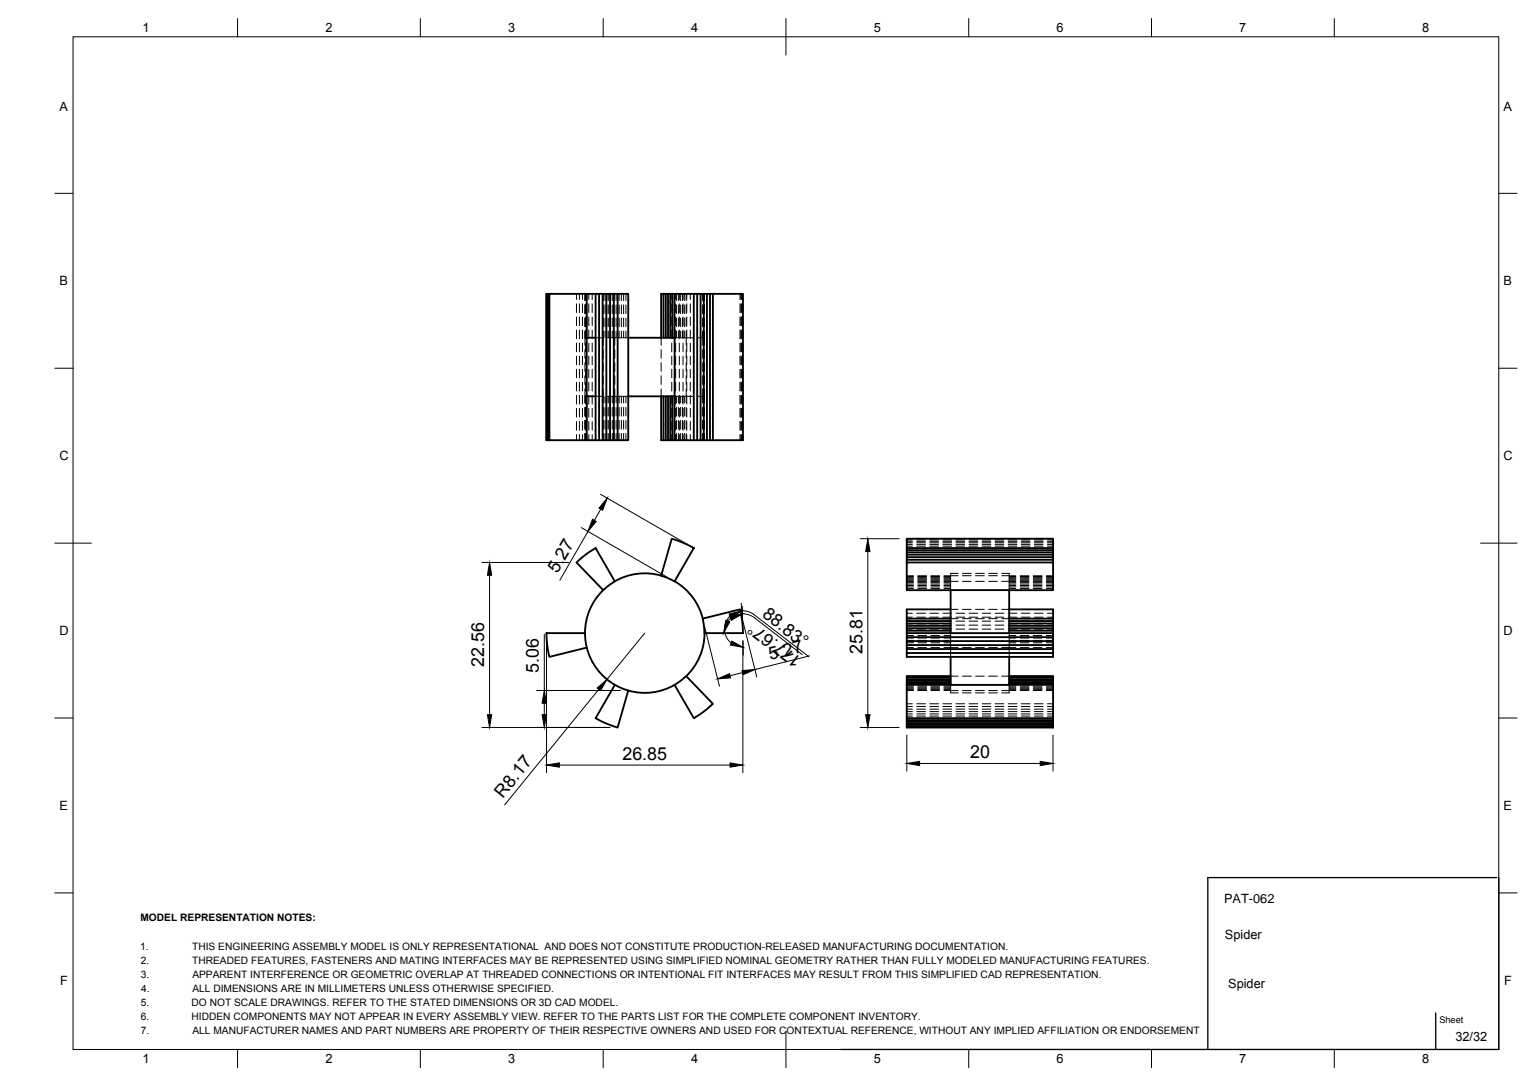
ISO-10303-21;
HEADER;
/* Generated by software containing ST-Developer
 * from STEP Tools, Inc. (www.steptools.com) 
 */

FILE_DESCRIPTION(
/* description */ ('Jaw-coupled motor to shaft test stand'),
/* implementation_level */ '2;1');

FILE_NAME(
/* name */ 'Spider.step',
/* time_stamp */ '2026-10-27T10:46:06-07:00',
/* author */ (''),
/* organization */ (''),
/* preprocessor_version */ 'ST-DEVELOPER v20.2',
/* originating_system */ 'Autodesk Translation Framework v15.17.0.0',
/* authorisation */ '');

FILE_SCHEMA (('AUTOMOTIVE_DESIGN { 1 0 10303 214 3 1 1 }'));
ENDSEC;

DATA;
#10=MECHANICAL_DESIGN_GEOMETRIC_PRESENTATION_REPRESENTATION('',(#369),#19361);
#304=SHAPE_REPRESENTATION_RELATIONSHIP('SRR','None',#19521,#336);
#336=ADVANCED_BREP_SHAPE_REPRESENTATION('',(#400),#19357);
#369=STYLED_ITEM('',(#19739),#400);
#400=MANIFOLD_SOLID_BREP('Body1',#11015);
#860=PLANE('',#12101);
#861=PLANE('',#12120);
#862=PLANE('',#12121);
#863=PLANE('',#12122);
#864=PLANE('',#12123);
#865=PLANE('',#12124);
#866=PLANE('',#12125);
#867=PLANE('',#12126);
#868=PLANE('',#12127);
#869=PLANE('',#12128);
#870=PLANE('',#12129);
#871=PLANE('',#12130);
#872=PLANE('',#12131);
#873=PLANE('',#12132);
#874=PLANE('',#12133);
#875=PLANE('',#12134);
#876=PLANE('',#12135);
#877=PLANE('',#12136);
#878=PLANE('',#12137);
#879=PLANE('',#12138);
#880=PLANE('',#12139);
#881=PLANE('',#12140);
#882=PLANE('',#12141);
#883=PLANE('',#12142);
#884=PLANE('',#12143);
#885=PLANE('',#12144);
#886=PLANE('',#12145);
#887=PLANE('',#12146);
#888=PLANE('',#12147);
#889=PLANE('',#12148);
#890=PLANE('',#12149);
#891=PLANE('',#12150);
#892=PLANE('',#12151);
#893=PLANE('',#12152);
#894=PLANE('',#12153);
#895=PLANE('',#12154);
#896=PLANE('',#12155);
#897=PLANE('',#12156);
#898=PLANE('',#12157);
#899=PLANE('',#12158);
#900=PLANE('',#12159);
#901=PLANE('',#12160);
#902=PLANE('',#12161);
#903=PLANE('',#12162);
#904=PLANE('',#12163);
#905=PLANE('',#12164);
#906=PLANE('',#12165);
#907=PLANE('',#12166);
#908=PLANE('',#12167);
#909=PLANE('',#12168);
#910=PLANE('',#12169);
#911=PLANE('',#12170);
#912=PLANE('',#12171);
#913=PLANE('',#12172);
#914=PLANE('',#12173);
#915=PLANE('',#12174);
#916=PLANE('',#12175);
#917=PLANE('',#12176);
#918=PLANE('',#12177);
#919=PLANE('',#12178);
#920=PLANE('',#12179);
#921=PLANE('',#12180);
#922=PLANE('',#12181);
#923=PLANE('',#12182);
#924=PLANE('',#12183);
#925=PLANE('',#12184);
#926=PLANE('',#12185);
#927=PLANE('',#12186);
#928=PLANE('',#12187);
#929=PLANE('',#12188);
#930=PLANE('',#12189);
#931=PLANE('',#12190);
#932=PLANE('',#12191);
#933=PLANE('',#12192);
#934=PLANE('',#12193);
#935=PLANE('',#12194);
#936=PLANE('',#12195);
#937=PLANE('',#12196);
#938=PLANE('',#12197);
#939=PLANE('',#12198);
#940=PLANE('',#12199);
#941=PLANE('',#12200);
#942=PLANE('',#12201);
#943=PLANE('',#12202);
#944=PLANE('',#12203);
#945=PLANE('',#12204);
#946=PLANE('',#12205);
#947=PLANE('',#12206);
#948=PLANE('',#12207);
#949=PLANE('',#12208);
#950=PLANE('',#12209);
#951=PLANE('',#12210);
#952=PLANE('',#12211);
#953=PLANE('',#12212);
#954=PLANE('',#12213);
#955=PLANE('',#12214);
#956=PLANE('',#12215);
#957=PLANE('',#12216);
#958=PLANE('',#12217);
#959=PLANE('',#12218);
#960=PLANE('',#12219);
#961=PLANE('',#12220);
#962=PLANE('',#12221);
#963=PLANE('',#12222);
#964=PLANE('',#12223);
#965=PLANE('',#12224);
#966=PLANE('',#12225);
#967=PLANE('',#12226);
#968=PLANE('',#12227);
#969=PLANE('',#12228);
#970=PLANE('',#12229);
#971=PLANE('',#12230);
#972=PLANE('',#12231);
#973=PLANE('',#12232);
#974=PLANE('',#12233);
#975=PLANE('',#12234);
#976=PLANE('',#12235);
#977=PLANE('',#12236);
#978=PLANE('',#12237);
#979=PLANE('',#12238);
#980=PLANE('',#12239);
#981=PLANE('',#12240);
#982=PLANE('',#12241);
#983=PLANE('',#12242);
#984=PLANE('',#12243);
#985=PLANE('',#12244);
#986=PLANE('',#12245);
#987=PLANE('',#12246);
#988=PLANE('',#12247);
#989=PLANE('',#12248);
#990=PLANE('',#12249);
#991=PLANE('',#12250);
#992=PLANE('',#12251);
#993=PLANE('',#12252);
#1459=FACE_OUTER_BOUND('',#2190,.T.);
#1460=FACE_OUTER_BOUND('',#2191,.T.);
#1461=FACE_OUTER_BOUND('',#2192,.T.);
#1462=FACE_OUTER_BOUND('',#2193,.T.);
#1463=FACE_OUTER_BOUND('',#2194,.T.);
#1464=FACE_OUTER_BOUND('',#2195,.T.);
#1465=FACE_OUTER_BOUND('',#2196,.T.);
#1466=FACE_OUTER_BOUND('',#2197,.T.);
#1467=FACE_OUTER_BOUND('',#2198,.T.);
#1468=FACE_OUTER_BOUND('',#2199,.T.);
#1469=FACE_OUTER_BOUND('',#2200,.T.);
#1470=FACE_OUTER_BOUND('',#2201,.T.);
#1471=FACE_OUTER_BOUND('',#2202,.T.);
#1472=FACE_OUTER_BOUND('',#2203,.T.);
#1473=FACE_OUTER_BOUND('',#2204,.T.);
#1474=FACE_OUTER_BOUND('',#2205,.T.);
#1475=FACE_OUTER_BOUND('',#2206,.T.);
#1476=FACE_OUTER_BOUND('',#2207,.T.);
#1477=FACE_OUTER_BOUND('',#2208,.T.);
#1478=FACE_OUTER_BOUND('',#2209,.T.);
#1479=FACE_OUTER_BOUND('',#2210,.T.);
#1480=FACE_OUTER_BOUND('',#2211,.T.);
#1481=FACE_OUTER_BOUND('',#2212,.T.);
#1482=FACE_OUTER_BOUND('',#2213,.T.);
#1483=FACE_OUTER_BOUND('',#2214,.T.);
#1484=FACE_OUTER_BOUND('',#2215,.T.);
#1485=FACE_OUTER_BOUND('',#2216,.T.);
#1486=FACE_OUTER_BOUND('',#2217,.T.);
#1487=FACE_OUTER_BOUND('',#2218,.T.);
#1488=FACE_OUTER_BOUND('',#2219,.T.);
#1489=FACE_OUTER_BOUND('',#2220,.T.);
#1490=FACE_OUTER_BOUND('',#2221,.T.);
#1491=FACE_OUTER_BOUND('',#2222,.T.);
#1492=FACE_OUTER_BOUND('',#2223,.T.);
#1493=FACE_OUTER_BOUND('',#2224,.T.);
#1494=FACE_OUTER_BOUND('',#2225,.T.);
#1495=FACE_OUTER_BOUND('',#2226,.T.);
#1496=FACE_OUTER_BOUND('',#2227,.T.);
#1497=FACE_OUTER_BOUND('',#2228,.T.);
#1498=FACE_OUTER_BOUND('',#2229,.T.);
#1499=FACE_OUTER_BOUND('',#2230,.T.);
#1500=FACE_OUTER_BOUND('',#2231,.T.);
#1501=FACE_OUTER_BOUND('',#2232,.T.);
#1502=FACE_OUTER_BOUND('',#2233,.T.);
#1503=FACE_OUTER_BOUND('',#2234,.T.);
#1504=FACE_OUTER_BOUND('',#2235,.T.);
#1505=FACE_OUTER_BOUND('',#2236,.T.);
#1506=FACE_OUTER_BOUND('',#2237,.T.);
#1507=FACE_OUTER_BOUND('',#2238,.T.);
#1508=FACE_OUTER_BOUND('',#2239,.T.);
#1509=FACE_OUTER_BOUND('',#2240,.T.);
#1510=FACE_OUTER_BOUND('',#2241,.T.);
#1511=FACE_OUTER_BOUND('',#2242,.T.);
#1512=FACE_OUTER_BOUND('',#2243,.T.);
#1513=FACE_OUTER_BOUND('',#2244,.T.);
#1514=FACE_OUTER_BOUND('',#2245,.T.);
#1515=FACE_OUTER_BOUND('',#2246,.T.);
#1516=FACE_OUTER_BOUND('',#2247,.T.);
#1517=FACE_OUTER_BOUND('',#2248,.T.);
#1518=FACE_OUTER_BOUND('',#2249,.T.);
#1519=FACE_OUTER_BOUND('',#2250,.T.);
#1520=FACE_OUTER_BOUND('',#2251,.T.);
#1521=FACE_OUTER_BOUND('',#2252,.T.);
#1522=FACE_OUTER_BOUND('',#2253,.T.);
#1523=FACE_OUTER_BOUND('',#2254,.T.);
#1524=FACE_OUTER_BOUND('',#2255,.T.);
#1525=FACE_OUTER_BOUND('',#2256,.T.);
#1526=FACE_OUTER_BOUND('',#2257,.T.);
#1527=FACE_OUTER_BOUND('',#2258,.T.);
#1528=FACE_OUTER_BOUND('',#2259,.T.);
#1529=FACE_OUTER_BOUND('',#2260,.T.);
#1530=FACE_OUTER_BOUND('',#2261,.T.);
#1531=FACE_OUTER_BOUND('',#2262,.T.);
#1532=FACE_OUTER_BOUND('',#2263,.T.);
#1533=FACE_OUTER_BOUND('',#2264,.T.);
#1534=FACE_OUTER_BOUND('',#2265,.T.);
#1535=FACE_OUTER_BOUND('',#2266,.T.);
#1536=FACE_OUTER_BOUND('',#2267,.T.);
#1537=FACE_OUTER_BOUND('',#2268,.T.);
#1538=FACE_OUTER_BOUND('',#2269,.T.);
#1539=FACE_OUTER_BOUND('',#2270,.T.);
#1540=FACE_OUTER_BOUND('',#2271,.T.);
#1541=FACE_OUTER_BOUND('',#2272,.T.);
#1542=FACE_OUTER_BOUND('',#2273,.T.);
#1543=FACE_OUTER_BOUND('',#2274,.T.);
#1544=FACE_OUTER_BOUND('',#2275,.T.);
#1545=FACE_OUTER_BOUND('',#2276,.T.);
#1546=FACE_OUTER_BOUND('',#2277,.T.);
#1547=FACE_OUTER_BOUND('',#2278,.T.);
#1548=FACE_OUTER_BOUND('',#2279,.T.);
#1549=FACE_OUTER_BOUND('',#2280,.T.);
#1550=FACE_OUTER_BOUND('',#2281,.T.);
#1551=FACE_OUTER_BOUND('',#2282,.T.);
#1552=FACE_OUTER_BOUND('',#2283,.T.);
#1553=FACE_OUTER_BOUND('',#2284,.T.);
#1554=FACE_OUTER_BOUND('',#2285,.T.);
#1555=FACE_OUTER_BOUND('',#2286,.T.);
#1556=FACE_OUTER_BOUND('',#2287,.T.);
#1557=FACE_OUTER_BOUND('',#2288,.T.);
#1558=FACE_OUTER_BOUND('',#2289,.T.);
#1559=FACE_OUTER_BOUND('',#2290,.T.);
#1560=FACE_OUTER_BOUND('',#2291,.T.);
#1561=FACE_OUTER_BOUND('',#2292,.T.);
#1562=FACE_OUTER_BOUND('',#2293,.T.);
#1563=FACE_OUTER_BOUND('',#2294,.T.);
#1564=FACE_OUTER_BOUND('',#2295,.T.);
#1565=FACE_OUTER_BOUND('',#2296,.T.);
#1566=FACE_OUTER_BOUND('',#2297,.T.);
#1567=FACE_OUTER_BOUND('',#2298,.T.);
#1568=FACE_OUTER_BOUND('',#2299,.T.);
#1569=FACE_OUTER_BOUND('',#2300,.T.);
#1570=FACE_OUTER_BOUND('',#2301,.T.);
#1571=FACE_OUTER_BOUND('',#2302,.T.);
#1572=FACE_OUTER_BOUND('',#2303,.T.);
#1573=FACE_OUTER_BOUND('',#2304,.T.);
#1574=FACE_OUTER_BOUND('',#2305,.T.);
#1575=FACE_OUTER_BOUND('',#2306,.T.);
#1576=FACE_OUTER_BOUND('',#2307,.T.);
#1577=FACE_OUTER_BOUND('',#2308,.T.);
#1578=FACE_OUTER_BOUND('',#2309,.T.);
#1579=FACE_OUTER_BOUND('',#2310,.T.);
#1580=FACE_OUTER_BOUND('',#2311,.T.);
#1581=FACE_OUTER_BOUND('',#2312,.T.);
#1582=FACE_OUTER_BOUND('',#2313,.T.);
#1583=FACE_OUTER_BOUND('',#2314,.T.);
#1584=FACE_OUTER_BOUND('',#2315,.T.);
#1585=FACE_OUTER_BOUND('',#2316,.T.);
#1586=FACE_OUTER_BOUND('',#2317,.T.);
#1587=FACE_OUTER_BOUND('',#2318,.T.);
#1588=FACE_OUTER_BOUND('',#2319,.T.);
#1589=FACE_OUTER_BOUND('',#2320,.T.);
#1590=FACE_OUTER_BOUND('',#2321,.T.);
#1591=FACE_OUTER_BOUND('',#2322,.T.);
#1592=FACE_OUTER_BOUND('',#2323,.T.);
#1593=FACE_OUTER_BOUND('',#2324,.T.);
#1594=FACE_OUTER_BOUND('',#2325,.T.);
#1595=FACE_OUTER_BOUND('',#2326,.T.);
#1596=FACE_OUTER_BOUND('',#2327,.T.);
#1597=FACE_OUTER_BOUND('',#2328,.T.);
#1598=FACE_OUTER_BOUND('',#2329,.T.);
#2190=EDGE_LOOP('',(#9272,#9273,#9274,#9275,#9276,#9277,#9278,#9279,#9280,
#9281,#9282,#9283,#9284,#9285,#9286,#9287,#9288,#9289,#9290,#9291,#9292,
#9293,#9294,#9295,#9296,#9297,#9298,#9299,#9300,#9301,#9302,#9303,#9304,
#9305,#9306,#9307,#9308,#9309,#9310,#9311,#9312,#9313,#9314,#9315,#9316,
#9317,#9318,#9319,#9320,#9321,#9322,#9323,#9324,#9325));
#2191=EDGE_LOOP('',(#9326,#9327,#9328,#9329));
#2192=EDGE_LOOP('',(#9330,#9331,#9332,#9333));
#2193=EDGE_LOOP('',(#9334,#9335,#9336,#9337));
#2194=EDGE_LOOP('',(#9338,#9339,#9340,#9341));
#2195=EDGE_LOOP('',(#9342,#9343,#9344,#9345));
#2196=EDGE_LOOP('',(#9346,#9347,#9348,#9349));
#2197=EDGE_LOOP('',(#9350,#9351,#9352,#9353,#9354,#9355,#9356,#9357,#9358,
#9359,#9360,#9361,#9362,#9363,#9364,#9365,#9366,#9367,#9368,#9369,#9370,
#9371,#9372,#9373,#9374,#9375,#9376,#9377,#9378,#9379,#9380,#9381,#9382,
#9383,#9384,#9385,#9386,#9387,#9388,#9389,#9390,#9391,#9392,#9393,#9394,
#9395,#9396,#9397,#9398,#9399,#9400,#9401,#9402,#9403));
#2198=EDGE_LOOP('',(#9404,#9405,#9406,#9407,#9408,#9409,#9410,#9411));
#2199=EDGE_LOOP('',(#9412,#9413,#9414,#9415));
#2200=EDGE_LOOP('',(#9416,#9417,#9418,#9419));
#2201=EDGE_LOOP('',(#9420,#9421,#9422,#9423));
#2202=EDGE_LOOP('',(#9424,#9425,#9426,#9427));
#2203=EDGE_LOOP('',(#9428,#9429,#9430,#9431));
#2204=EDGE_LOOP('',(#9432,#9433,#9434,#9435));
#2205=EDGE_LOOP('',(#9436,#9437,#9438,#9439));
#2206=EDGE_LOOP('',(#9440,#9441,#9442,#9443,#9444,#9445,#9446,#9447,#9448,
#9449,#9450,#9451,#9452,#9453));
#2207=EDGE_LOOP('',(#9454,#9455,#9456,#9457));
#2208=EDGE_LOOP('',(#9458,#9459,#9460,#9461));
#2209=EDGE_LOOP('',(#9462,#9463,#9464,#9465));
#2210=EDGE_LOOP('',(#9466,#9467,#9468,#9469));
#2211=EDGE_LOOP('',(#9470,#9471,#9472,#9473));
#2212=EDGE_LOOP('',(#9474,#9475,#9476,#9477));
#2213=EDGE_LOOP('',(#9478,#9479,#9480,#9481));
#2214=EDGE_LOOP('',(#9482,#9483,#9484,#9485));
#2215=EDGE_LOOP('',(#9486,#9487,#9488,#9489));
#2216=EDGE_LOOP('',(#9490,#9491,#9492,#9493));
#2217=EDGE_LOOP('',(#9494,#9495,#9496,#9497));
#2218=EDGE_LOOP('',(#9498,#9499,#9500,#9501,#9502,#9503,#9504,#9505));
#2219=EDGE_LOOP('',(#9506,#9507,#9508,#9509,#9510,#9511,#9512,#9513,#9514,
#9515,#9516,#9517,#9518,#9519));
#2220=EDGE_LOOP('',(#9520,#9521,#9522,#9523,#9524,#9525,#9526,#9527));
#2221=EDGE_LOOP('',(#9528,#9529,#9530,#9531));
#2222=EDGE_LOOP('',(#9532,#9533,#9534,#9535));
#2223=EDGE_LOOP('',(#9536,#9537,#9538,#9539));
#2224=EDGE_LOOP('',(#9540,#9541,#9542,#9543));
#2225=EDGE_LOOP('',(#9544,#9545,#9546,#9547));
#2226=EDGE_LOOP('',(#9548,#9549,#9550,#9551));
#2227=EDGE_LOOP('',(#9552,#9553,#9554,#9555));
#2228=EDGE_LOOP('',(#9556,#9557,#9558,#9559,#9560,#9561,#9562,#9563,#9564,
#9565,#9566,#9567,#9568,#9569));
#2229=EDGE_LOOP('',(#9570,#9571,#9572,#9573));
#2230=EDGE_LOOP('',(#9574,#9575,#9576,#9577));
#2231=EDGE_LOOP('',(#9578,#9579,#9580,#9581));
#2232=EDGE_LOOP('',(#9582,#9583,#9584,#9585));
#2233=EDGE_LOOP('',(#9586,#9587,#9588,#9589));
#2234=EDGE_LOOP('',(#9590,#9591,#9592,#9593));
#2235=EDGE_LOOP('',(#9594,#9595,#9596,#9597));
#2236=EDGE_LOOP('',(#9598,#9599,#9600,#9601));
#2237=EDGE_LOOP('',(#9602,#9603,#9604,#9605));
#2238=EDGE_LOOP('',(#9606,#9607,#9608,#9609));
#2239=EDGE_LOOP('',(#9610,#9611,#9612,#9613));
#2240=EDGE_LOOP('',(#9614,#9615,#9616,#9617,#9618,#9619,#9620,#9621));
#2241=EDGE_LOOP('',(#9622,#9623,#9624,#9625,#9626,#9627,#9628,#9629,#9630,
#9631,#9632,#9633,#9634,#9635));
#2242=EDGE_LOOP('',(#9636,#9637,#9638,#9639,#9640,#9641,#9642,#9643));
#2243=EDGE_LOOP('',(#9644,#9645,#9646,#9647));
#2244=EDGE_LOOP('',(#9648,#9649,#9650,#9651));
#2245=EDGE_LOOP('',(#9652,#9653,#9654,#9655));
#2246=EDGE_LOOP('',(#9656,#9657,#9658,#9659));
#2247=EDGE_LOOP('',(#9660,#9661,#9662,#9663));
#2248=EDGE_LOOP('',(#9664,#9665,#9666,#9667));
#2249=EDGE_LOOP('',(#9668,#9669,#9670,#9671));
#2250=EDGE_LOOP('',(#9672,#9673,#9674,#9675,#9676,#9677,#9678,#9679,#9680,
#9681,#9682,#9683,#9684,#9685));
#2251=EDGE_LOOP('',(#9686,#9687,#9688,#9689));
#2252=EDGE_LOOP('',(#9690,#9691,#9692,#9693));
#2253=EDGE_LOOP('',(#9694,#9695,#9696,#9697));
#2254=EDGE_LOOP('',(#9698,#9699,#9700,#9701));
#2255=EDGE_LOOP('',(#9702,#9703,#9704,#9705));
#2256=EDGE_LOOP('',(#9706,#9707,#9708,#9709));
#2257=EDGE_LOOP('',(#9710,#9711,#9712,#9713));
#2258=EDGE_LOOP('',(#9714,#9715,#9716,#9717));
#2259=EDGE_LOOP('',(#9718,#9719,#9720,#9721));
#2260=EDGE_LOOP('',(#9722,#9723,#9724,#9725));
#2261=EDGE_LOOP('',(#9726,#9727,#9728,#9729));
#2262=EDGE_LOOP('',(#9730,#9731,#9732,#9733,#9734,#9735,#9736,#9737));
#2263=EDGE_LOOP('',(#9738,#9739,#9740,#9741,#9742,#9743,#9744,#9745,#9746,
#9747,#9748,#9749,#9750,#9751));
#2264=EDGE_LOOP('',(#9752,#9753,#9754,#9755,#9756,#9757,#9758,#9759));
#2265=EDGE_LOOP('',(#9760,#9761,#9762,#9763));
#2266=EDGE_LOOP('',(#9764,#9765,#9766,#9767));
#2267=EDGE_LOOP('',(#9768,#9769,#9770,#9771));
#2268=EDGE_LOOP('',(#9772,#9773,#9774,#9775));
#2269=EDGE_LOOP('',(#9776,#9777,#9778,#9779));
#2270=EDGE_LOOP('',(#9780,#9781,#9782,#9783));
#2271=EDGE_LOOP('',(#9784,#9785,#9786,#9787));
#2272=EDGE_LOOP('',(#9788,#9789,#9790,#9791,#9792,#9793,#9794,#9795,#9796,
#9797,#9798,#9799,#9800,#9801));
#2273=EDGE_LOOP('',(#9802,#9803,#9804,#9805));
#2274=EDGE_LOOP('',(#9806,#9807,#9808,#9809));
#2275=EDGE_LOOP('',(#9810,#9811,#9812,#9813));
#2276=EDGE_LOOP('',(#9814,#9815,#9816,#9817));
#2277=EDGE_LOOP('',(#9818,#9819,#9820,#9821));
#2278=EDGE_LOOP('',(#9822,#9823,#9824,#9825));
#2279=EDGE_LOOP('',(#9826,#9827,#9828,#9829));
#2280=EDGE_LOOP('',(#9830,#9831,#9832,#9833));
#2281=EDGE_LOOP('',(#9834,#9835,#9836,#9837));
#2282=EDGE_LOOP('',(#9838,#9839,#9840,#9841));
#2283=EDGE_LOOP('',(#9842,#9843,#9844,#9845));
#2284=EDGE_LOOP('',(#9846,#9847,#9848,#9849,#9850,#9851,#9852,#9853));
#2285=EDGE_LOOP('',(#9854,#9855,#9856,#9857,#9858,#9859,#9860,#9861,#9862,
#9863,#9864,#9865,#9866,#9867));
#2286=EDGE_LOOP('',(#9868,#9869,#9870,#9871,#9872,#9873,#9874,#9875));
#2287=EDGE_LOOP('',(#9876,#9877,#9878,#9879));
#2288=EDGE_LOOP('',(#9880,#9881,#9882,#9883));
#2289=EDGE_LOOP('',(#9884,#9885,#9886,#9887));
#2290=EDGE_LOOP('',(#9888,#9889,#9890,#9891));
#2291=EDGE_LOOP('',(#9892,#9893,#9894,#9895));
#2292=EDGE_LOOP('',(#9896,#9897,#9898,#9899));
#2293=EDGE_LOOP('',(#9900,#9901,#9902,#9903));
#2294=EDGE_LOOP('',(#9904,#9905,#9906,#9907,#9908,#9909,#9910,#9911,#9912,
#9913,#9914,#9915,#9916,#9917));
#2295=EDGE_LOOP('',(#9918,#9919,#9920,#9921));
#2296=EDGE_LOOP('',(#9922,#9923,#9924,#9925));
#2297=EDGE_LOOP('',(#9926,#9927,#9928,#9929));
#2298=EDGE_LOOP('',(#9930,#9931,#9932,#9933));
#2299=EDGE_LOOP('',(#9934,#9935,#9936,#9937));
#2300=EDGE_LOOP('',(#9938,#9939,#9940,#9941));
#2301=EDGE_LOOP('',(#9942,#9943,#9944,#9945));
#2302=EDGE_LOOP('',(#9946,#9947,#9948,#9949));
#2303=EDGE_LOOP('',(#9950,#9951,#9952,#9953));
#2304=EDGE_LOOP('',(#9954,#9955,#9956,#9957));
#2305=EDGE_LOOP('',(#9958,#9959,#9960,#9961));
#2306=EDGE_LOOP('',(#9962,#9963,#9964,#9965,#9966,#9967,#9968,#9969));
#2307=EDGE_LOOP('',(#9970,#9971,#9972,#9973,#9974,#9975,#9976,#9977,#9978,
#9979,#9980,#9981,#9982,#9983));
#2308=EDGE_LOOP('',(#9984,#9985,#9986,#9987,#9988,#9989,#9990,#9991));
#2309=EDGE_LOOP('',(#9992,#9993,#9994,#9995));
#2310=EDGE_LOOP('',(#9996,#9997,#9998,#9999));
#2311=EDGE_LOOP('',(#10000,#10001,#10002,#10003));
#2312=EDGE_LOOP('',(#10004,#10005,#10006,#10007));
#2313=EDGE_LOOP('',(#10008,#10009,#10010,#10011));
#2314=EDGE_LOOP('',(#10012,#10013,#10014,#10015));
#2315=EDGE_LOOP('',(#10016,#10017,#10018,#10019));
#2316=EDGE_LOOP('',(#10020,#10021,#10022,#10023,#10024,#10025,#10026,#10027,
#10028,#10029,#10030,#10031,#10032,#10033));
#2317=EDGE_LOOP('',(#10034,#10035,#10036,#10037));
#2318=EDGE_LOOP('',(#10038,#10039,#10040,#10041));
#2319=EDGE_LOOP('',(#10042,#10043,#10044,#10045));
#2320=EDGE_LOOP('',(#10046,#10047,#10048,#10049));
#2321=EDGE_LOOP('',(#10050,#10051,#10052,#10053));
#2322=EDGE_LOOP('',(#10054,#10055,#10056,#10057));
#2323=EDGE_LOOP('',(#10058,#10059,#10060,#10061));
#2324=EDGE_LOOP('',(#10062,#10063,#10064,#10065));
#2325=EDGE_LOOP('',(#10066,#10067,#10068,#10069));
#2326=EDGE_LOOP('',(#10070,#10071,#10072,#10073));
#2327=EDGE_LOOP('',(#10074,#10075,#10076,#10077));
#2328=EDGE_LOOP('',(#10078,#10079,#10080,#10081,#10082,#10083,#10084,#10085));
#2329=EDGE_LOOP('',(#10086,#10087,#10088,#10089,#10090,#10091,#10092,#10093,
#10094,#10095,#10096,#10097,#10098,#10099));
#3061=LINE('',#18255,#4214);
#3062=LINE('',#18257,#4215);
#3063=LINE('',#18259,#4216);
#3064=LINE('',#18261,#4217);
#3065=LINE('',#18263,#4218);
#3066=LINE('',#18265,#4219);
#3067=LINE('',#18267,#4220);
#3068=LINE('',#18269,#4221);
#3069=LINE('',#18273,#4222);
#3070=LINE('',#18275,#4223);
#3071=LINE('',#18277,#4224);
#3072=LINE('',#18279,#4225);
#3073=LINE('',#18281,#4226);
#3074=LINE('',#18283,#4227);
#3075=LINE('',#18285,#4228);
#3076=LINE('',#18287,#4229);
#3077=LINE('',#18291,#4230);
#3078=LINE('',#18293,#4231);
#3079=LINE('',#18295,#4232);
#3080=LINE('',#18297,#4233);
#3081=LINE('',#18299,#4234);
#3082=LINE('',#18301,#4235);
#3083=LINE('',#18303,#4236);
#3084=LINE('',#18305,#4237);
#3085=LINE('',#18309,#4238);
#3086=LINE('',#18311,#4239);
#3087=LINE('',#18313,#4240);
#3088=LINE('',#18315,#4241);
#3089=LINE('',#18317,#4242);
#3090=LINE('',#18319,#4243);
#3091=LINE('',#18321,#4244);
#3092=LINE('',#18323,#4245);
#3093=LINE('',#18327,#4246);
#3094=LINE('',#18329,#4247);
#3095=LINE('',#18331,#4248);
#3096=LINE('',#18333,#4249);
#3097=LINE('',#18335,#4250);
#3098=LINE('',#18337,#4251);
#3099=LINE('',#18339,#4252);
#3100=LINE('',#18341,#4253);
#3101=LINE('',#18345,#4254);
#3102=LINE('',#18347,#4255);
#3103=LINE('',#18349,#4256);
#3104=LINE('',#18351,#4257);
#3105=LINE('',#18353,#4258);
#3106=LINE('',#18355,#4259);
#3107=LINE('',#18357,#4260);
#3108=LINE('',#18359,#4261);
#3109=LINE('',#18363,#4262);
#3110=LINE('',#18366,#4263);
#3111=LINE('',#18369,#4264);
#3112=LINE('',#18372,#4265);
#3113=LINE('',#18375,#4266);
#3114=LINE('',#18378,#4267);
#3115=LINE('',#18381,#4268);
#3116=LINE('',#18383,#4269);
#3117=LINE('',#18387,#4270);
#3118=LINE('',#18389,#4271);
#3119=LINE('',#18393,#4272);
#3120=LINE('',#18395,#4273);
#3121=LINE('',#18399,#4274);
#3122=LINE('',#18401,#4275);
#3123=LINE('',#18403,#4276);
#3124=LINE('',#18405,#4277);
#3125=LINE('',#18407,#4278);
#3126=LINE('',#18409,#4279);
#3127=LINE('',#18411,#4280);
#3128=LINE('',#18413,#4281);
#3129=LINE('',#18414,#4282);
#3130=LINE('',#18416,#4283);
#3131=LINE('',#18418,#4284);
#3132=LINE('',#18420,#4285);
#3133=LINE('',#18422,#4286);
#3134=LINE('',#18424,#4287);
#3135=LINE('',#18426,#4288);
#3136=LINE('',#18428,#4289);
#3137=LINE('',#18429,#4290);
#3138=LINE('',#18431,#4291);
#3139=LINE('',#18433,#4292);
#3140=LINE('',#18435,#4293);
#3141=LINE('',#18437,#4294);
#3142=LINE('',#18439,#4295);
#3143=LINE('',#18441,#4296);
#3144=LINE('',#18443,#4297);
#3145=LINE('',#18444,#4298);
#3146=LINE('',#18446,#4299);
#3147=LINE('',#18448,#4300);
#3148=LINE('',#18450,#4301);
#3149=LINE('',#18452,#4302);
#3150=LINE('',#18454,#4303);
#3151=LINE('',#18456,#4304);
#3152=LINE('',#18458,#4305);
#3153=LINE('',#18459,#4306);
#3154=LINE('',#18461,#4307);
#3155=LINE('',#18463,#4308);
#3156=LINE('',#18465,#4309);
#3157=LINE('',#18467,#4310);
#3158=LINE('',#18469,#4311);
#3159=LINE('',#18471,#4312);
#3160=LINE('',#18473,#4313);
#3161=LINE('',#18474,#4314);
#3162=LINE('',#18476,#4315);
#3163=LINE('',#18478,#4316);
#3164=LINE('',#18480,#4317);
#3165=LINE('',#18482,#4318);
#3166=LINE('',#18484,#4319);
#3167=LINE('',#18486,#4320);
#3168=LINE('',#18487,#4321);
#3169=LINE('',#18490,#4322);
#3170=LINE('',#18492,#4323);
#3171=LINE('',#18494,#4324);
#3172=LINE('',#18496,#4325);
#3173=LINE('',#18497,#4326);
#3174=LINE('',#18500,#4327);
#3175=LINE('',#18501,#4328);
#3176=LINE('',#18504,#4329);
#3177=LINE('',#18505,#4330);
#3178=LINE('',#18508,#4331);
#3179=LINE('',#18509,#4332);
#3180=LINE('',#18512,#4333);
#3181=LINE('',#18513,#4334);
#3182=LINE('',#18516,#4335);
#3183=LINE('',#18517,#4336);
#3184=LINE('',#18520,#4337);
#3185=LINE('',#18521,#4338);
#3186=LINE('',#18524,#4339);
#3187=LINE('',#18525,#4340);
#3188=LINE('',#18529,#4341);
#3189=LINE('',#18531,#4342);
#3190=LINE('',#18533,#4343);
#3191=LINE('',#18535,#4344);
#3192=LINE('',#18537,#4345);
#3193=LINE('',#18538,#4346);
#3194=LINE('',#18540,#4347);
#3195=LINE('',#18542,#4348);
#3196=LINE('',#18544,#4349);
#3197=LINE('',#18546,#4350);
#3198=LINE('',#18548,#4351);
#3199=LINE('',#18549,#4352);
#3200=LINE('',#18551,#4353);
#3201=LINE('',#18552,#4354);
#3202=LINE('',#18554,#4355);
#3203=LINE('',#18556,#4356);
#3204=LINE('',#18558,#4357);
#3205=LINE('',#18562,#4358);
#3206=LINE('',#18563,#4359);
#3207=LINE('',#18566,#4360);
#3208=LINE('',#18567,#4361);
#3209=LINE('',#18570,#4362);
#3210=LINE('',#18571,#4363);
#3211=LINE('',#18574,#4364);
#3212=LINE('',#18575,#4365);
#3213=LINE('',#18578,#4366);
#3214=LINE('',#18579,#4367);
#3215=LINE('',#18582,#4368);
#3216=LINE('',#18583,#4369);
#3217=LINE('',#18585,#4370);
#3218=LINE('',#18589,#4371);
#3219=LINE('',#18591,#4372);
#3220=LINE('',#18593,#4373);
#3221=LINE('',#18595,#4374);
#3222=LINE('',#18596,#4375);
#3223=LINE('',#18599,#4376);
#3224=LINE('',#18600,#4377);
#3225=LINE('',#18603,#4378);
#3226=LINE('',#18604,#4379);
#3227=LINE('',#18607,#4380);
#3228=LINE('',#18608,#4381);
#3229=LINE('',#18611,#4382);
#3230=LINE('',#18612,#4383);
#3231=LINE('',#18615,#4384);
#3232=LINE('',#18616,#4385);
#3233=LINE('',#18619,#4386);
#3234=LINE('',#18620,#4387);
#3235=LINE('',#18623,#4388);
#3236=LINE('',#18624,#4389);
#3237=LINE('',#18628,#4390);
#3238=LINE('',#18630,#4391);
#3239=LINE('',#18632,#4392);
#3240=LINE('',#18634,#4393);
#3241=LINE('',#18636,#4394);
#3242=LINE('',#18637,#4395);
#3243=LINE('',#18639,#4396);
#3244=LINE('',#18641,#4397);
#3245=LINE('',#18643,#4398);
#3246=LINE('',#18645,#4399);
#3247=LINE('',#18647,#4400);
#3248=LINE('',#18648,#4401);
#3249=LINE('',#18650,#4402);
#3250=LINE('',#18651,#4403);
#3251=LINE('',#18653,#4404);
#3252=LINE('',#18655,#4405);
#3253=LINE('',#18657,#4406);
#3254=LINE('',#18661,#4407);
#3255=LINE('',#18662,#4408);
#3256=LINE('',#18665,#4409);
#3257=LINE('',#18666,#4410);
#3258=LINE('',#18669,#4411);
#3259=LINE('',#18670,#4412);
#3260=LINE('',#18673,#4413);
#3261=LINE('',#18674,#4414);
#3262=LINE('',#18677,#4415);
#3263=LINE('',#18678,#4416);
#3264=LINE('',#18681,#4417);
#3265=LINE('',#18682,#4418);
#3266=LINE('',#18684,#4419);
#3267=LINE('',#18688,#4420);
#3268=LINE('',#18690,#4421);
#3269=LINE('',#18692,#4422);
#3270=LINE('',#18694,#4423);
#3271=LINE('',#18695,#4424);
#3272=LINE('',#18698,#4425);
#3273=LINE('',#18699,#4426);
#3274=LINE('',#18702,#4427);
#3275=LINE('',#18703,#4428);
#3276=LINE('',#18706,#4429);
#3277=LINE('',#18707,#4430);
#3278=LINE('',#18710,#4431);
#3279=LINE('',#18711,#4432);
#3280=LINE('',#18714,#4433);
#3281=LINE('',#18715,#4434);
#3282=LINE('',#18718,#4435);
#3283=LINE('',#18719,#4436);
#3284=LINE('',#18722,#4437);
#3285=LINE('',#18723,#4438);
#3286=LINE('',#18727,#4439);
#3287=LINE('',#18729,#4440);
#3288=LINE('',#18731,#4441);
#3289=LINE('',#18733,#4442);
#3290=LINE('',#18735,#4443);
#3291=LINE('',#18736,#4444);
#3292=LINE('',#18738,#4445);
#3293=LINE('',#18740,#4446);
#3294=LINE('',#18742,#4447);
#3295=LINE('',#18744,#4448);
#3296=LINE('',#18746,#4449);
#3297=LINE('',#18747,#4450);
#3298=LINE('',#18749,#4451);
#3299=LINE('',#18750,#4452);
#3300=LINE('',#18752,#4453);
#3301=LINE('',#18754,#4454);
#3302=LINE('',#18756,#4455);
#3303=LINE('',#18760,#4456);
#3304=LINE('',#18761,#4457);
#3305=LINE('',#18764,#4458);
#3306=LINE('',#18765,#4459);
#3307=LINE('',#18768,#4460);
#3308=LINE('',#18769,#4461);
#3309=LINE('',#18772,#4462);
#3310=LINE('',#18773,#4463);
#3311=LINE('',#18776,#4464);
#3312=LINE('',#18777,#4465);
#3313=LINE('',#18780,#4466);
#3314=LINE('',#18781,#4467);
#3315=LINE('',#18783,#4468);
#3316=LINE('',#18787,#4469);
#3317=LINE('',#18789,#4470);
#3318=LINE('',#18791,#4471);
#3319=LINE('',#18793,#4472);
#3320=LINE('',#18794,#4473);
#3321=LINE('',#18797,#4474);
#3322=LINE('',#18798,#4475);
#3323=LINE('',#18801,#4476);
#3324=LINE('',#18802,#4477);
#3325=LINE('',#18805,#4478);
#3326=LINE('',#18806,#4479);
#3327=LINE('',#18809,#4480);
#3328=LINE('',#18810,#4481);
#3329=LINE('',#18813,#4482);
#3330=LINE('',#18814,#4483);
#3331=LINE('',#18817,#4484);
#3332=LINE('',#18818,#4485);
#3333=LINE('',#18821,#4486);
#3334=LINE('',#18822,#4487);
#3335=LINE('',#18826,#4488);
#3336=LINE('',#18828,#4489);
#3337=LINE('',#18830,#4490);
#3338=LINE('',#18832,#4491);
#3339=LINE('',#18834,#4492);
#3340=LINE('',#18835,#4493);
#3341=LINE('',#18837,#4494);
#3342=LINE('',#18839,#4495);
#3343=LINE('',#18841,#4496);
#3344=LINE('',#18843,#4497);
#3345=LINE('',#18845,#4498);
#3346=LINE('',#18846,#4499);
#3347=LINE('',#18848,#4500);
#3348=LINE('',#18849,#4501);
#3349=LINE('',#18851,#4502);
#3350=LINE('',#18853,#4503);
#3351=LINE('',#18855,#4504);
#3352=LINE('',#18859,#4505);
#3353=LINE('',#18860,#4506);
#3354=LINE('',#18863,#4507);
#3355=LINE('',#18864,#4508);
#3356=LINE('',#18867,#4509);
#3357=LINE('',#18868,#4510);
#3358=LINE('',#18871,#4511);
#3359=LINE('',#18872,#4512);
#3360=LINE('',#18875,#4513);
#3361=LINE('',#18876,#4514);
#3362=LINE('',#18879,#4515);
#3363=LINE('',#18880,#4516);
#3364=LINE('',#18882,#4517);
#3365=LINE('',#18886,#4518);
#3366=LINE('',#18888,#4519);
#3367=LINE('',#18890,#4520);
#3368=LINE('',#18892,#4521);
#3369=LINE('',#18893,#4522);
#3370=LINE('',#18896,#4523);
#3371=LINE('',#18897,#4524);
#3372=LINE('',#18900,#4525);
#3373=LINE('',#18901,#4526);
#3374=LINE('',#18904,#4527);
#3375=LINE('',#18905,#4528);
#3376=LINE('',#18908,#4529);
#3377=LINE('',#18909,#4530);
#3378=LINE('',#18912,#4531);
#3379=LINE('',#18913,#4532);
#3380=LINE('',#18916,#4533);
#3381=LINE('',#18917,#4534);
#3382=LINE('',#18920,#4535);
#3383=LINE('',#18921,#4536);
#3384=LINE('',#18925,#4537);
#3385=LINE('',#18927,#4538);
#3386=LINE('',#18929,#4539);
#3387=LINE('',#18931,#4540);
#3388=LINE('',#18933,#4541);
#3389=LINE('',#18934,#4542);
#3390=LINE('',#18936,#4543);
#3391=LINE('',#18938,#4544);
#3392=LINE('',#18940,#4545);
#3393=LINE('',#18942,#4546);
#3394=LINE('',#18944,#4547);
#3395=LINE('',#18945,#4548);
#3396=LINE('',#18947,#4549);
#3397=LINE('',#18948,#4550);
#3398=LINE('',#18950,#4551);
#3399=LINE('',#18952,#4552);
#3400=LINE('',#18954,#4553);
#3401=LINE('',#18958,#4554);
#3402=LINE('',#18959,#4555);
#3403=LINE('',#18962,#4556);
#3404=LINE('',#18963,#4557);
#3405=LINE('',#18966,#4558);
#3406=LINE('',#18967,#4559);
#3407=LINE('',#18970,#4560);
#3408=LINE('',#18971,#4561);
#3409=LINE('',#18974,#4562);
#3410=LINE('',#18975,#4563);
#3411=LINE('',#18978,#4564);
#3412=LINE('',#18979,#4565);
#3413=LINE('',#18981,#4566);
#3414=LINE('',#18985,#4567);
#3415=LINE('',#18987,#4568);
#3416=LINE('',#18989,#4569);
#3417=LINE('',#18991,#4570);
#3418=LINE('',#18992,#4571);
#3419=LINE('',#18995,#4572);
#3420=LINE('',#18996,#4573);
#3421=LINE('',#18999,#4574);
#3422=LINE('',#19000,#4575);
#3423=LINE('',#19003,#4576);
#3424=LINE('',#19004,#4577);
#3425=LINE('',#19007,#4578);
#3426=LINE('',#19008,#4579);
#3427=LINE('',#19011,#4580);
#3428=LINE('',#19012,#4581);
#3429=LINE('',#19015,#4582);
#3430=LINE('',#19016,#4583);
#3431=LINE('',#19019,#4584);
#3432=LINE('',#19020,#4585);
#3433=LINE('',#19024,#4586);
#3434=LINE('',#19026,#4587);
#3435=LINE('',#19028,#4588);
#3436=LINE('',#19030,#4589);
#3437=LINE('',#19032,#4590);
#3438=LINE('',#19033,#4591);
#3439=LINE('',#19035,#4592);
#3440=LINE('',#19037,#4593);
#3441=LINE('',#19039,#4594);
#3442=LINE('',#19041,#4595);
#3443=LINE('',#19043,#4596);
#3444=LINE('',#19044,#4597);
#3445=LINE('',#19046,#4598);
#3446=LINE('',#19047,#4599);
#3447=LINE('',#19049,#4600);
#3448=LINE('',#19051,#4601);
#3449=LINE('',#19053,#4602);
#3450=LINE('',#19057,#4603);
#3451=LINE('',#19058,#4604);
#3452=LINE('',#19061,#4605);
#3453=LINE('',#19062,#4606);
#3454=LINE('',#19065,#4607);
#3455=LINE('',#19066,#4608);
#3456=LINE('',#19069,#4609);
#3457=LINE('',#19070,#4610);
#3458=LINE('',#19073,#4611);
#3459=LINE('',#19074,#4612);
#3460=LINE('',#19077,#4613);
#3461=LINE('',#19078,#4614);
#3462=LINE('',#19080,#4615);
#4214=VECTOR('',#14484,1.);
#4215=VECTOR('',#14485,1.);
#4216=VECTOR('',#14486,1.);
#4217=VECTOR('',#14487,1.);
#4218=VECTOR('',#14488,1.);
#4219=VECTOR('',#14489,1.);
#4220=VECTOR('',#14490,1.);
#4221=VECTOR('',#14491,1.);
#4222=VECTOR('',#14494,1.);
#4223=VECTOR('',#14495,1.);
#4224=VECTOR('',#14496,1.);
#4225=VECTOR('',#14497,1.);
#4226=VECTOR('',#14498,1.);
#4227=VECTOR('',#14499,1.);
#4228=VECTOR('',#14500,1.);
#4229=VECTOR('',#14501,1.);
#4230=VECTOR('',#14504,1.);
#4231=VECTOR('',#14505,1.);
#4232=VECTOR('',#14506,1.);
#4233=VECTOR('',#14507,1.);
#4234=VECTOR('',#14508,1.);
#4235=VECTOR('',#14509,1.);
#4236=VECTOR('',#14510,1.);
#4237=VECTOR('',#14511,1.);
#4238=VECTOR('',#14514,1.);
#4239=VECTOR('',#14515,1.);
#4240=VECTOR('',#14516,1.);
#4241=VECTOR('',#14517,1.);
#4242=VECTOR('',#14518,1.);
#4243=VECTOR('',#14519,1.);
#4244=VECTOR('',#14520,1.);
#4245=VECTOR('',#14521,1.);
#4246=VECTOR('',#14524,1.);
#4247=VECTOR('',#14525,1.);
#4248=VECTOR('',#14526,1.);
#4249=VECTOR('',#14527,1.);
#4250=VECTOR('',#14528,1.);
#4251=VECTOR('',#14529,1.);
#4252=VECTOR('',#14530,1.);
#4253=VECTOR('',#14531,1.);
#4254=VECTOR('',#14534,1.);
#4255=VECTOR('',#14535,1.);
#4256=VECTOR('',#14536,1.);
#4257=VECTOR('',#14537,1.);
#4258=VECTOR('',#14538,1.);
#4259=VECTOR('',#14539,1.);
#4260=VECTOR('',#14540,1.);
#4261=VECTOR('',#14541,1.);
#4262=VECTOR('',#14546,1.);
#4263=VECTOR('',#14549,1.);
#4264=VECTOR('',#14552,1.);
#4265=VECTOR('',#14555,1.);
#4266=VECTOR('',#14558,1.);
#4267=VECTOR('',#14561,1.);
#4268=VECTOR('',#14564,1.);
#4269=VECTOR('',#14565,1.);
#4270=VECTOR('',#14570,1.);
#4271=VECTOR('',#14571,1.);
#4272=VECTOR('',#14576,1.);
#4273=VECTOR('',#14577,1.);
#4274=VECTOR('',#14582,1.);
#4275=VECTOR('',#14583,1.);
#4276=VECTOR('',#14584,1.);
#4277=VECTOR('',#14585,1.);
#4278=VECTOR('',#14586,1.);
#4279=VECTOR('',#14587,1.);
#4280=VECTOR('',#14588,1.);
#4281=VECTOR('',#14589,1.);
#4282=VECTOR('',#14590,1.);
#4283=VECTOR('',#14591,1.);
#4284=VECTOR('',#14592,1.);
#4285=VECTOR('',#14593,1.);
#4286=VECTOR('',#14594,1.);
#4287=VECTOR('',#14595,1.);
#4288=VECTOR('',#14596,1.);
#4289=VECTOR('',#14597,1.);
#4290=VECTOR('',#14598,1.);
#4291=VECTOR('',#14599,1.);
#4292=VECTOR('',#14600,1.);
#4293=VECTOR('',#14601,1.);
#4294=VECTOR('',#14602,1.);
#4295=VECTOR('',#14603,1.);
#4296=VECTOR('',#14604,1.);
#4297=VECTOR('',#14605,1.);
#4298=VECTOR('',#14606,1.);
#4299=VECTOR('',#14607,1.);
#4300=VECTOR('',#14608,1.);
#4301=VECTOR('',#14609,1.);
#4302=VECTOR('',#14610,1.);
#4303=VECTOR('',#14611,1.);
#4304=VECTOR('',#14612,1.);
#4305=VECTOR('',#14613,1.);
#4306=VECTOR('',#14614,1.);
#4307=VECTOR('',#14615,1.);
#4308=VECTOR('',#14616,1.);
#4309=VECTOR('',#14617,1.);
#4310=VECTOR('',#14618,1.);
#4311=VECTOR('',#14619,1.);
#4312=VECTOR('',#14620,1.);
#4313=VECTOR('',#14621,1.);
#4314=VECTOR('',#14622,1.);
#4315=VECTOR('',#14623,1.);
#4316=VECTOR('',#14624,1.);
#4317=VECTOR('',#14625,1.);
#4318=VECTOR('',#14626,1.);
#4319=VECTOR('',#14627,1.);
#4320=VECTOR('',#14628,1.);
#4321=VECTOR('',#14629,1.);
#4322=VECTOR('',#14632,1.);
#4323=VECTOR('',#14633,1.);
#4324=VECTOR('',#14634,1.);
#4325=VECTOR('',#14635,1.);
#4326=VECTOR('',#14636,1.);
#4327=VECTOR('',#14639,1.);
#4328=VECTOR('',#14640,1.);
#4329=VECTOR('',#14643,1.);
#4330=VECTOR('',#14644,1.);
#4331=VECTOR('',#14647,1.);
#4332=VECTOR('',#14648,1.);
#4333=VECTOR('',#14651,1.);
#4334=VECTOR('',#14652,1.);
#4335=VECTOR('',#14655,1.);
#4336=VECTOR('',#14656,1.);
#4337=VECTOR('',#14659,1.);
#4338=VECTOR('',#14660,1.);
#4339=VECTOR('',#14663,1.);
#4340=VECTOR('',#14664,1.);
#4341=VECTOR('',#14667,1.);
#4342=VECTOR('',#14668,1.);
#4343=VECTOR('',#14669,1.);
#4344=VECTOR('',#14670,1.);
#4345=VECTOR('',#14671,1.);
#4346=VECTOR('',#14672,1.);
#4347=VECTOR('',#14673,1.);
#4348=VECTOR('',#14674,1.);
#4349=VECTOR('',#14675,1.);
#4350=VECTOR('',#14676,1.);
#4351=VECTOR('',#14677,1.);
#4352=VECTOR('',#14678,1.);
#4353=VECTOR('',#14681,1.);
#4354=VECTOR('',#14682,1.);
#4355=VECTOR('',#14685,1.);
#4356=VECTOR('',#14688,1.);
#4357=VECTOR('',#14691,1.);
#4358=VECTOR('',#14696,1.);
#4359=VECTOR('',#14697,1.);
#4360=VECTOR('',#14700,1.);
#4361=VECTOR('',#14701,1.);
#4362=VECTOR('',#14704,1.);
#4363=VECTOR('',#14705,1.);
#4364=VECTOR('',#14708,1.);
#4365=VECTOR('',#14709,1.);
#4366=VECTOR('',#14712,1.);
#4367=VECTOR('',#14713,1.);
#4368=VECTOR('',#14716,1.);
#4369=VECTOR('',#14717,1.);
#4370=VECTOR('',#14720,1.);
#4371=VECTOR('',#14725,1.);
#4372=VECTOR('',#14726,1.);
#4373=VECTOR('',#14727,1.);
#4374=VECTOR('',#14728,1.);
#4375=VECTOR('',#14729,1.);
#4376=VECTOR('',#14732,1.);
#4377=VECTOR('',#14733,1.);
#4378=VECTOR('',#14736,1.);
#4379=VECTOR('',#14737,1.);
#4380=VECTOR('',#14740,1.);
#4381=VECTOR('',#14741,1.);
#4382=VECTOR('',#14744,1.);
#4383=VECTOR('',#14745,1.);
#4384=VECTOR('',#14748,1.);
#4385=VECTOR('',#14749,1.);
#4386=VECTOR('',#14752,1.);
#4387=VECTOR('',#14753,1.);
#4388=VECTOR('',#14756,1.);
#4389=VECTOR('',#14757,1.);
#4390=VECTOR('',#14760,1.);
#4391=VECTOR('',#14761,1.);
#4392=VECTOR('',#14762,1.);
#4393=VECTOR('',#14763,1.);
#4394=VECTOR('',#14764,1.);
#4395=VECTOR('',#14765,1.);
#4396=VECTOR('',#14766,1.);
#4397=VECTOR('',#14767,1.);
#4398=VECTOR('',#14768,1.);
#4399=VECTOR('',#14769,1.);
#4400=VECTOR('',#14770,1.);
#4401=VECTOR('',#14771,1.);
#4402=VECTOR('',#14774,1.);
#4403=VECTOR('',#14775,1.);
#4404=VECTOR('',#14778,1.);
#4405=VECTOR('',#14781,1.);
#4406=VECTOR('',#14784,1.);
#4407=VECTOR('',#14789,1.);
#4408=VECTOR('',#14790,1.);
#4409=VECTOR('',#14793,1.);
#4410=VECTOR('',#14794,1.);
#4411=VECTOR('',#14797,1.);
#4412=VECTOR('',#14798,1.);
#4413=VECTOR('',#14801,1.);
#4414=VECTOR('',#14802,1.);
#4415=VECTOR('',#14805,1.);
#4416=VECTOR('',#14806,1.);
#4417=VECTOR('',#14809,1.);
#4418=VECTOR('',#14810,1.);
#4419=VECTOR('',#14813,1.);
#4420=VECTOR('',#14818,1.);
#4421=VECTOR('',#14819,1.);
#4422=VECTOR('',#14820,1.);
#4423=VECTOR('',#14821,1.);
#4424=VECTOR('',#14822,1.);
#4425=VECTOR('',#14825,1.);
#4426=VECTOR('',#14826,1.);
#4427=VECTOR('',#14829,1.);
#4428=VECTOR('',#14830,1.);
#4429=VECTOR('',#14833,1.);
#4430=VECTOR('',#14834,1.);
#4431=VECTOR('',#14837,1.);
#4432=VECTOR('',#14838,1.);
#4433=VECTOR('',#14841,1.);
#4434=VECTOR('',#14842,1.);
#4435=VECTOR('',#14845,1.);
#4436=VECTOR('',#14846,1.);
#4437=VECTOR('',#14849,1.);
#4438=VECTOR('',#14850,1.);
#4439=VECTOR('',#14853,1.);
#4440=VECTOR('',#14854,1.);
#4441=VECTOR('',#14855,1.);
#4442=VECTOR('',#14856,1.);
#4443=VECTOR('',#14857,1.);
#4444=VECTOR('',#14858,1.);
#4445=VECTOR('',#14859,1.);
#4446=VECTOR('',#14860,1.);
#4447=VECTOR('',#14861,1.);
#4448=VECTOR('',#14862,1.);
#4449=VECTOR('',#14863,1.);
#4450=VECTOR('',#14864,1.);
#4451=VECTOR('',#14867,1.);
#4452=VECTOR('',#14868,1.);
#4453=VECTOR('',#14871,1.);
#4454=VECTOR('',#14874,1.);
#4455=VECTOR('',#14877,1.);
#4456=VECTOR('',#14882,1.);
#4457=VECTOR('',#14883,1.);
#4458=VECTOR('',#14886,1.);
#4459=VECTOR('',#14887,1.);
#4460=VECTOR('',#14890,1.);
#4461=VECTOR('',#14891,1.);
#4462=VECTOR('',#14894,1.);
#4463=VECTOR('',#14895,1.);
#4464=VECTOR('',#14898,1.);
#4465=VECTOR('',#14899,1.);
#4466=VECTOR('',#14902,1.);
#4467=VECTOR('',#14903,1.);
#4468=VECTOR('',#14906,1.);
#4469=VECTOR('',#14911,1.);
#4470=VECTOR('',#14912,1.);
#4471=VECTOR('',#14913,1.);
#4472=VECTOR('',#14914,1.);
#4473=VECTOR('',#14915,1.);
#4474=VECTOR('',#14918,1.);
#4475=VECTOR('',#14919,1.);
#4476=VECTOR('',#14922,1.);
#4477=VECTOR('',#14923,1.);
#4478=VECTOR('',#14926,1.);
#4479=VECTOR('',#14927,1.);
#4480=VECTOR('',#14930,1.);
#4481=VECTOR('',#14931,1.);
#4482=VECTOR('',#14934,1.);
#4483=VECTOR('',#14935,1.);
#4484=VECTOR('',#14938,1.);
#4485=VECTOR('',#14939,1.);
#4486=VECTOR('',#14942,1.);
#4487=VECTOR('',#14943,1.);
#4488=VECTOR('',#14946,1.);
#4489=VECTOR('',#14947,1.);
#4490=VECTOR('',#14948,1.);
#4491=VECTOR('',#14949,1.);
#4492=VECTOR('',#14950,1.);
#4493=VECTOR('',#14951,1.);
#4494=VECTOR('',#14952,1.);
#4495=VECTOR('',#14953,1.);
#4496=VECTOR('',#14954,1.);
#4497=VECTOR('',#14955,1.);
#4498=VECTOR('',#14956,1.);
#4499=VECTOR('',#14957,1.);
#4500=VECTOR('',#14960,1.);
#4501=VECTOR('',#14961,1.);
#4502=VECTOR('',#14964,1.);
#4503=VECTOR('',#14967,1.);
#4504=VECTOR('',#14970,1.);
#4505=VECTOR('',#14975,1.);
#4506=VECTOR('',#14976,1.);
#4507=VECTOR('',#14979,1.);
#4508=VECTOR('',#14980,1.);
#4509=VECTOR('',#14983,1.);
#4510=VECTOR('',#14984,1.);
#4511=VECTOR('',#14987,1.);
#4512=VECTOR('',#14988,1.);
#4513=VECTOR('',#14991,1.);
#4514=VECTOR('',#14992,1.);
#4515=VECTOR('',#14995,1.);
#4516=VECTOR('',#14996,1.);
#4517=VECTOR('',#14999,1.);
#4518=VECTOR('',#15004,1.);
#4519=VECTOR('',#15005,1.);
#4520=VECTOR('',#15006,1.);
#4521=VECTOR('',#15007,1.);
#4522=VECTOR('',#15008,1.);
#4523=VECTOR('',#15011,1.);
#4524=VECTOR('',#15012,1.);
#4525=VECTOR('',#15015,1.);
#4526=VECTOR('',#15016,1.);
#4527=VECTOR('',#15019,1.);
#4528=VECTOR('',#15020,1.);
#4529=VECTOR('',#15023,1.);
#4530=VECTOR('',#15024,1.);
#4531=VECTOR('',#15027,1.);
#4532=VECTOR('',#15028,1.);
#4533=VECTOR('',#15031,1.);
#4534=VECTOR('',#15032,1.);
#4535=VECTOR('',#15035,1.);
#4536=VECTOR('',#15036,1.);
#4537=VECTOR('',#15039,1.);
#4538=VECTOR('',#15040,1.);
#4539=VECTOR('',#15041,1.);
#4540=VECTOR('',#15042,1.);
#4541=VECTOR('',#15043,1.);
#4542=VECTOR('',#15044,1.);
#4543=VECTOR('',#15045,1.);
#4544=VECTOR('',#15046,1.);
#4545=VECTOR('',#15047,1.);
#4546=VECTOR('',#15048,1.);
#4547=VECTOR('',#15049,1.);
#4548=VECTOR('',#15050,1.);
#4549=VECTOR('',#15053,1.);
#4550=VECTOR('',#15054,1.);
#4551=VECTOR('',#15057,1.);
#4552=VECTOR('',#15060,1.);
#4553=VECTOR('',#15063,1.);
#4554=VECTOR('',#15068,1.);
#4555=VECTOR('',#15069,1.);
#4556=VECTOR('',#15072,1.);
#4557=VECTOR('',#15073,1.);
#4558=VECTOR('',#15076,1.);
#4559=VECTOR('',#15077,1.);
#4560=VECTOR('',#15080,1.);
#4561=VECTOR('',#15081,1.);
#4562=VECTOR('',#15084,1.);
#4563=VECTOR('',#15085,1.);
#4564=VECTOR('',#15088,1.);
#4565=VECTOR('',#15089,1.);
#4566=VECTOR('',#15092,1.);
#4567=VECTOR('',#15097,1.);
#4568=VECTOR('',#15098,1.);
#4569=VECTOR('',#15099,1.);
#4570=VECTOR('',#15100,1.);
#4571=VECTOR('',#15101,1.);
#4572=VECTOR('',#15104,1.);
#4573=VECTOR('',#15105,1.);
#4574=VECTOR('',#15108,1.);
#4575=VECTOR('',#15109,1.);
#4576=VECTOR('',#15112,1.);
#4577=VECTOR('',#15113,1.);
#4578=VECTOR('',#15116,1.);
#4579=VECTOR('',#15117,1.);
#4580=VECTOR('',#15120,1.);
#4581=VECTOR('',#15121,1.);
#4582=VECTOR('',#15124,1.);
#4583=VECTOR('',#15125,1.);
#4584=VECTOR('',#15128,1.);
#4585=VECTOR('',#15129,1.);
#4586=VECTOR('',#15132,1.);
#4587=VECTOR('',#15133,1.);
#4588=VECTOR('',#15134,1.);
#4589=VECTOR('',#15135,1.);
#4590=VECTOR('',#15136,1.);
#4591=VECTOR('',#15137,1.);
#4592=VECTOR('',#15138,1.);
#4593=VECTOR('',#15139,1.);
#4594=VECTOR('',#15140,1.);
#4595=VECTOR('',#15141,1.);
#4596=VECTOR('',#15142,1.);
#4597=VECTOR('',#15143,1.);
#4598=VECTOR('',#15146,1.);
#4599=VECTOR('',#15147,1.);
#4600=VECTOR('',#15150,1.);
#4601=VECTOR('',#15153,1.);
#4602=VECTOR('',#15156,1.);
#4603=VECTOR('',#15161,1.);
#4604=VECTOR('',#15162,1.);
#4605=VECTOR('',#15165,1.);
#4606=VECTOR('',#15166,1.);
#4607=VECTOR('',#15169,1.);
#4608=VECTOR('',#15170,1.);
#4609=VECTOR('',#15173,1.);
#4610=VECTOR('',#15174,1.);
#4611=VECTOR('',#15177,1.);
#4612=VECTOR('',#15178,1.);
#4613=VECTOR('',#15181,1.);
#4614=VECTOR('',#15182,1.);
#4615=VECTOR('',#15185,1.);
#4911=CIRCLE('',#12102,0.817);
#4912=CIRCLE('',#12103,0.817);
#4913=CIRCLE('',#12104,0.817);
#4914=CIRCLE('',#12105,0.817);
#4915=CIRCLE('',#12106,0.817);
#4916=CIRCLE('',#12107,0.817);
#4917=CIRCLE('',#12109,0.817);
#4918=CIRCLE('',#12111,0.817);
#4919=CIRCLE('',#12113,0.817);
#4920=CIRCLE('',#12115,0.817);
#4921=CIRCLE('',#12117,0.817);
#4922=CIRCLE('',#12119,0.817);
#5556=VERTEX_POINT('',#18253);
#5557=VERTEX_POINT('',#18254);
#5558=VERTEX_POINT('',#18256);
#5559=VERTEX_POINT('',#18258);
#5560=VERTEX_POINT('',#18260);
#5561=VERTEX_POINT('',#18262);
#5562=VERTEX_POINT('',#18264);
#5563=VERTEX_POINT('',#18266);
#5564=VERTEX_POINT('',#18268);
#5565=VERTEX_POINT('',#18270);
#5566=VERTEX_POINT('',#18272);
#5567=VERTEX_POINT('',#18274);
#5568=VERTEX_POINT('',#18276);
#5569=VERTEX_POINT('',#18278);
#5570=VERTEX_POINT('',#18280);
#5571=VERTEX_POINT('',#18282);
#5572=VERTEX_POINT('',#18284);
#5573=VERTEX_POINT('',#18286);
#5574=VERTEX_POINT('',#18288);
#5575=VERTEX_POINT('',#18290);
#5576=VERTEX_POINT('',#18292);
#5577=VERTEX_POINT('',#18294);
#5578=VERTEX_POINT('',#18296);
#5579=VERTEX_POINT('',#18298);
#5580=VERTEX_POINT('',#18300);
#5581=VERTEX_POINT('',#18302);
#5582=VERTEX_POINT('',#18304);
#5583=VERTEX_POINT('',#18306);
#5584=VERTEX_POINT('',#18308);
#5585=VERTEX_POINT('',#18310);
#5586=VERTEX_POINT('',#18312);
#5587=VERTEX_POINT('',#18314);
#5588=VERTEX_POINT('',#18316);
#5589=VERTEX_POINT('',#18318);
#5590=VERTEX_POINT('',#18320);
#5591=VERTEX_POINT('',#18322);
#5592=VERTEX_POINT('',#18324);
#5593=VERTEX_POINT('',#18326);
#5594=VERTEX_POINT('',#18328);
#5595=VERTEX_POINT('',#18330);
#5596=VERTEX_POINT('',#18332);
#5597=VERTEX_POINT('',#18334);
#5598=VERTEX_POINT('',#18336);
#5599=VERTEX_POINT('',#18338);
#5600=VERTEX_POINT('',#18340);
#5601=VERTEX_POINT('',#18342);
#5602=VERTEX_POINT('',#18344);
#5603=VERTEX_POINT('',#18346);
#5604=VERTEX_POINT('',#18348);
#5605=VERTEX_POINT('',#18350);
#5606=VERTEX_POINT('',#18352);
#5607=VERTEX_POINT('',#18354);
#5608=VERTEX_POINT('',#18356);
#5609=VERTEX_POINT('',#18358);
#5610=VERTEX_POINT('',#18362);
#5611=VERTEX_POINT('',#18364);
#5612=VERTEX_POINT('',#18368);
#5613=VERTEX_POINT('',#18370);
#5614=VERTEX_POINT('',#18374);
#5615=VERTEX_POINT('',#18376);
#5616=VERTEX_POINT('',#18380);
#5617=VERTEX_POINT('',#18382);
#5618=VERTEX_POINT('',#18386);
#5619=VERTEX_POINT('',#18388);
#5620=VERTEX_POINT('',#18392);
#5621=VERTEX_POINT('',#18394);
#5622=VERTEX_POINT('',#18398);
#5623=VERTEX_POINT('',#18400);
#5624=VERTEX_POINT('',#18402);
#5625=VERTEX_POINT('',#18404);
#5626=VERTEX_POINT('',#18406);
#5627=VERTEX_POINT('',#18408);
#5628=VERTEX_POINT('',#18410);
#5629=VERTEX_POINT('',#18412);
#5630=VERTEX_POINT('',#18415);
#5631=VERTEX_POINT('',#18417);
#5632=VERTEX_POINT('',#18419);
#5633=VERTEX_POINT('',#18421);
#5634=VERTEX_POINT('',#18423);
#5635=VERTEX_POINT('',#18425);
#5636=VERTEX_POINT('',#18427);
#5637=VERTEX_POINT('',#18430);
#5638=VERTEX_POINT('',#18432);
#5639=VERTEX_POINT('',#18434);
#5640=VERTEX_POINT('',#18436);
#5641=VERTEX_POINT('',#18438);
#5642=VERTEX_POINT('',#18440);
#5643=VERTEX_POINT('',#18442);
#5644=VERTEX_POINT('',#18445);
#5645=VERTEX_POINT('',#18447);
#5646=VERTEX_POINT('',#18449);
#5647=VERTEX_POINT('',#18451);
#5648=VERTEX_POINT('',#18453);
#5649=VERTEX_POINT('',#18455);
#5650=VERTEX_POINT('',#18457);
#5651=VERTEX_POINT('',#18460);
#5652=VERTEX_POINT('',#18462);
#5653=VERTEX_POINT('',#18464);
#5654=VERTEX_POINT('',#18466);
#5655=VERTEX_POINT('',#18468);
#5656=VERTEX_POINT('',#18470);
#5657=VERTEX_POINT('',#18472);
#5658=VERTEX_POINT('',#18475);
#5659=VERTEX_POINT('',#18477);
#5660=VERTEX_POINT('',#18479);
#5661=VERTEX_POINT('',#18481);
#5662=VERTEX_POINT('',#18483);
#5663=VERTEX_POINT('',#18485);
#5664=VERTEX_POINT('',#18489);
#5665=VERTEX_POINT('',#18491);
#5666=VERTEX_POINT('',#18493);
#5667=VERTEX_POINT('',#18495);
#5668=VERTEX_POINT('',#18499);
#5669=VERTEX_POINT('',#18503);
#5670=VERTEX_POINT('',#18507);
#5671=VERTEX_POINT('',#18511);
#5672=VERTEX_POINT('',#18515);
#5673=VERTEX_POINT('',#18519);
#5674=VERTEX_POINT('',#18523);
#5675=VERTEX_POINT('',#18527);
#5676=VERTEX_POINT('',#18528);
#5677=VERTEX_POINT('',#18530);
#5678=VERTEX_POINT('',#18532);
#5679=VERTEX_POINT('',#18534);
#5680=VERTEX_POINT('',#18536);
#5681=VERTEX_POINT('',#18539);
#5682=VERTEX_POINT('',#18541);
#5683=VERTEX_POINT('',#18543);
#5684=VERTEX_POINT('',#18545);
#5685=VERTEX_POINT('',#18547);
#5686=VERTEX_POINT('',#18561);
#5687=VERTEX_POINT('',#18565);
#5688=VERTEX_POINT('',#18569);
#5689=VERTEX_POINT('',#18573);
#5690=VERTEX_POINT('',#18577);
#5691=VERTEX_POINT('',#18581);
#5692=VERTEX_POINT('',#18588);
#5693=VERTEX_POINT('',#18590);
#5694=VERTEX_POINT('',#18592);
#5695=VERTEX_POINT('',#18594);
#5696=VERTEX_POINT('',#18598);
#5697=VERTEX_POINT('',#18602);
#5698=VERTEX_POINT('',#18606);
#5699=VERTEX_POINT('',#18610);
#5700=VERTEX_POINT('',#18614);
#5701=VERTEX_POINT('',#18618);
#5702=VERTEX_POINT('',#18622);
#5703=VERTEX_POINT('',#18626);
#5704=VERTEX_POINT('',#18627);
#5705=VERTEX_POINT('',#18629);
#5706=VERTEX_POINT('',#18631);
#5707=VERTEX_POINT('',#18633);
#5708=VERTEX_POINT('',#18635);
#5709=VERTEX_POINT('',#18638);
#5710=VERTEX_POINT('',#18640);
#5711=VERTEX_POINT('',#18642);
#5712=VERTEX_POINT('',#18644);
#5713=VERTEX_POINT('',#18646);
#5714=VERTEX_POINT('',#18660);
#5715=VERTEX_POINT('',#18664);
#5716=VERTEX_POINT('',#18668);
#5717=VERTEX_POINT('',#18672);
#5718=VERTEX_POINT('',#18676);
#5719=VERTEX_POINT('',#18680);
#5720=VERTEX_POINT('',#18687);
#5721=VERTEX_POINT('',#18689);
#5722=VERTEX_POINT('',#18691);
#5723=VERTEX_POINT('',#18693);
#5724=VERTEX_POINT('',#18697);
#5725=VERTEX_POINT('',#18701);
#5726=VERTEX_POINT('',#18705);
#5727=VERTEX_POINT('',#18709);
#5728=VERTEX_POINT('',#18713);
#5729=VERTEX_POINT('',#18717);
#5730=VERTEX_POINT('',#18721);
#5731=VERTEX_POINT('',#18725);
#5732=VERTEX_POINT('',#18726);
#5733=VERTEX_POINT('',#18728);
#5734=VERTEX_POINT('',#18730);
#5735=VERTEX_POINT('',#18732);
#5736=VERTEX_POINT('',#18734);
#5737=VERTEX_POINT('',#18737);
#5738=VERTEX_POINT('',#18739);
#5739=VERTEX_POINT('',#18741);
#5740=VERTEX_POINT('',#18743);
#5741=VERTEX_POINT('',#18745);
#5742=VERTEX_POINT('',#18759);
#5743=VERTEX_POINT('',#18763);
#5744=VERTEX_POINT('',#18767);
#5745=VERTEX_POINT('',#18771);
#5746=VERTEX_POINT('',#18775);
#5747=VERTEX_POINT('',#18779);
#5748=VERTEX_POINT('',#18786);
#5749=VERTEX_POINT('',#18788);
#5750=VERTEX_POINT('',#18790);
#5751=VERTEX_POINT('',#18792);
#5752=VERTEX_POINT('',#18796);
#5753=VERTEX_POINT('',#18800);
#5754=VERTEX_POINT('',#18804);
#5755=VERTEX_POINT('',#18808);
#5756=VERTEX_POINT('',#18812);
#5757=VERTEX_POINT('',#18816);
#5758=VERTEX_POINT('',#18820);
#5759=VERTEX_POINT('',#18824);
#5760=VERTEX_POINT('',#18825);
#5761=VERTEX_POINT('',#18827);
#5762=VERTEX_POINT('',#18829);
#5763=VERTEX_POINT('',#18831);
#5764=VERTEX_POINT('',#18833);
#5765=VERTEX_POINT('',#18836);
#5766=VERTEX_POINT('',#18838);
#5767=VERTEX_POINT('',#18840);
#5768=VERTEX_POINT('',#18842);
#5769=VERTEX_POINT('',#18844);
#5770=VERTEX_POINT('',#18858);
#5771=VERTEX_POINT('',#18862);
#5772=VERTEX_POINT('',#18866);
#5773=VERTEX_POINT('',#18870);
#5774=VERTEX_POINT('',#18874);
#5775=VERTEX_POINT('',#18878);
#5776=VERTEX_POINT('',#18885);
#5777=VERTEX_POINT('',#18887);
#5778=VERTEX_POINT('',#18889);
#5779=VERTEX_POINT('',#18891);
#5780=VERTEX_POINT('',#18895);
#5781=VERTEX_POINT('',#18899);
#5782=VERTEX_POINT('',#18903);
#5783=VERTEX_POINT('',#18907);
#5784=VERTEX_POINT('',#18911);
#5785=VERTEX_POINT('',#18915);
#5786=VERTEX_POINT('',#18919);
#5787=VERTEX_POINT('',#18923);
#5788=VERTEX_POINT('',#18924);
#5789=VERTEX_POINT('',#18926);
#5790=VERTEX_POINT('',#18928);
#5791=VERTEX_POINT('',#18930);
#5792=VERTEX_POINT('',#18932);
#5793=VERTEX_POINT('',#18935);
#5794=VERTEX_POINT('',#18937);
#5795=VERTEX_POINT('',#18939);
#5796=VERTEX_POINT('',#18941);
#5797=VERTEX_POINT('',#18943);
#5798=VERTEX_POINT('',#18957);
#5799=VERTEX_POINT('',#18961);
#5800=VERTEX_POINT('',#18965);
#5801=VERTEX_POINT('',#18969);
#5802=VERTEX_POINT('',#18973);
#5803=VERTEX_POINT('',#18977);
#5804=VERTEX_POINT('',#18984);
#5805=VERTEX_POINT('',#18986);
#5806=VERTEX_POINT('',#18988);
#5807=VERTEX_POINT('',#18990);
#5808=VERTEX_POINT('',#18994);
#5809=VERTEX_POINT('',#18998);
#5810=VERTEX_POINT('',#19002);
#5811=VERTEX_POINT('',#19006);
#5812=VERTEX_POINT('',#19010);
#5813=VERTEX_POINT('',#19014);
#5814=VERTEX_POINT('',#19018);
#5815=VERTEX_POINT('',#19022);
#5816=VERTEX_POINT('',#19023);
#5817=VERTEX_POINT('',#19025);
#5818=VERTEX_POINT('',#19027);
#5819=VERTEX_POINT('',#19029);
#5820=VERTEX_POINT('',#19031);
#5821=VERTEX_POINT('',#19034);
#5822=VERTEX_POINT('',#19036);
#5823=VERTEX_POINT('',#19038);
#5824=VERTEX_POINT('',#19040);
#5825=VERTEX_POINT('',#19042);
#5826=VERTEX_POINT('',#19056);
#5827=VERTEX_POINT('',#19060);
#5828=VERTEX_POINT('',#19064);
#5829=VERTEX_POINT('',#19068);
#5830=VERTEX_POINT('',#19072);
#5831=VERTEX_POINT('',#19076);
#6847=EDGE_CURVE('',#5556,#5557,#3061,.T.);
#6848=EDGE_CURVE('',#5558,#5556,#3062,.T.);
#6849=EDGE_CURVE('',#5559,#5558,#3063,.T.);
#6850=EDGE_CURVE('',#5560,#5559,#3064,.T.);
#6851=EDGE_CURVE('',#5561,#5560,#3065,.T.);
#6852=EDGE_CURVE('',#5562,#5561,#3066,.T.);
#6853=EDGE_CURVE('',#5563,#5562,#3067,.T.);
#6854=EDGE_CURVE('',#5564,#5563,#3068,.T.);
#6855=EDGE_CURVE('',#5564,#5565,#4911,.T.);
#6856=EDGE_CURVE('',#5566,#5565,#3069,.T.);
#6857=EDGE_CURVE('',#5567,#5566,#3070,.T.);
#6858=EDGE_CURVE('',#5568,#5567,#3071,.T.);
#6859=EDGE_CURVE('',#5569,#5568,#3072,.T.);
#6860=EDGE_CURVE('',#5570,#5569,#3073,.T.);
#6861=EDGE_CURVE('',#5571,#5570,#3074,.T.);
#6862=EDGE_CURVE('',#5572,#5571,#3075,.T.);
#6863=EDGE_CURVE('',#5573,#5572,#3076,.T.);
#6864=EDGE_CURVE('',#5573,#5574,#4912,.T.);
#6865=EDGE_CURVE('',#5575,#5574,#3077,.T.);
#6866=EDGE_CURVE('',#5576,#5575,#3078,.T.);
#6867=EDGE_CURVE('',#5577,#5576,#3079,.T.);
#6868=EDGE_CURVE('',#5578,#5577,#3080,.T.);
#6869=EDGE_CURVE('',#5579,#5578,#3081,.T.);
#6870=EDGE_CURVE('',#5580,#5579,#3082,.T.);
#6871=EDGE_CURVE('',#5581,#5580,#3083,.T.);
#6872=EDGE_CURVE('',#5582,#5581,#3084,.T.);
#6873=EDGE_CURVE('',#5582,#5583,#4913,.T.);
#6874=EDGE_CURVE('',#5584,#5583,#3085,.T.);
#6875=EDGE_CURVE('',#5585,#5584,#3086,.T.);
#6876=EDGE_CURVE('',#5586,#5585,#3087,.T.);
#6877=EDGE_CURVE('',#5587,#5586,#3088,.T.);
#6878=EDGE_CURVE('',#5588,#5587,#3089,.T.);
#6879=EDGE_CURVE('',#5589,#5588,#3090,.T.);
#6880=EDGE_CURVE('',#5590,#5589,#3091,.T.);
#6881=EDGE_CURVE('',#5591,#5590,#3092,.T.);
#6882=EDGE_CURVE('',#5591,#5592,#4914,.T.);
#6883=EDGE_CURVE('',#5593,#5592,#3093,.T.);
#6884=EDGE_CURVE('',#5594,#5593,#3094,.T.);
#6885=EDGE_CURVE('',#5595,#5594,#3095,.T.);
#6886=EDGE_CURVE('',#5596,#5595,#3096,.T.);
#6887=EDGE_CURVE('',#5597,#5596,#3097,.T.);
#6888=EDGE_CURVE('',#5598,#5597,#3098,.T.);
#6889=EDGE_CURVE('',#5599,#5598,#3099,.T.);
#6890=EDGE_CURVE('',#5600,#5599,#3100,.T.);
#6891=EDGE_CURVE('',#5600,#5601,#4915,.T.);
#6892=EDGE_CURVE('',#5602,#5601,#3101,.T.);
#6893=EDGE_CURVE('',#5603,#5602,#3102,.T.);
#6894=EDGE_CURVE('',#5604,#5603,#3103,.T.);
#6895=EDGE_CURVE('',#5605,#5604,#3104,.T.);
#6896=EDGE_CURVE('',#5606,#5605,#3105,.T.);
#6897=EDGE_CURVE('',#5607,#5606,#3106,.T.);
#6898=EDGE_CURVE('',#5608,#5607,#3107,.T.);
#6899=EDGE_CURVE('',#5609,#5608,#3108,.T.);
#6900=EDGE_CURVE('',#5609,#5557,#4916,.T.);
#6901=EDGE_CURVE('',#5610,#5600,#3109,.T.);
#6902=EDGE_CURVE('',#5611,#5610,#4917,.T.);
#6903=EDGE_CURVE('',#5601,#5611,#3110,.T.);
#6904=EDGE_CURVE('',#5612,#5564,#3111,.T.);
#6905=EDGE_CURVE('',#5613,#5612,#4918,.T.);
#6906=EDGE_CURVE('',#5565,#5613,#3112,.T.);
#6907=EDGE_CURVE('',#5614,#5582,#3113,.T.);
#6908=EDGE_CURVE('',#5615,#5614,#4919,.T.);
#6909=EDGE_CURVE('',#5583,#5615,#3114,.T.);
#6910=EDGE_CURVE('',#5592,#5616,#3115,.T.);
#6911=EDGE_CURVE('',#5617,#5591,#3116,.T.);
#6912=EDGE_CURVE('',#5616,#5617,#4920,.T.);
#6913=EDGE_CURVE('',#5574,#5618,#3117,.T.);
#6914=EDGE_CURVE('',#5619,#5573,#3118,.T.);
#6915=EDGE_CURVE('',#5618,#5619,#4921,.T.);
#6916=EDGE_CURVE('',#5557,#5620,#3119,.T.);
#6917=EDGE_CURVE('',#5621,#5609,#3120,.T.);
#6918=EDGE_CURVE('',#5620,#5621,#4922,.T.);
#6919=EDGE_CURVE('',#5620,#5622,#3121,.T.);
#6920=EDGE_CURVE('',#5623,#5621,#3122,.T.);
#6921=EDGE_CURVE('',#5624,#5623,#3123,.T.);
#6922=EDGE_CURVE('',#5625,#5624,#3124,.T.);
#6923=EDGE_CURVE('',#5626,#5625,#3125,.T.);
#6924=EDGE_CURVE('',#5627,#5626,#3126,.T.);
#6925=EDGE_CURVE('',#5628,#5627,#3127,.T.);
#6926=EDGE_CURVE('',#5629,#5628,#3128,.T.);
#6927=EDGE_CURVE('',#5611,#5629,#3129,.T.);
#6928=EDGE_CURVE('',#5630,#5610,#3130,.T.);
#6929=EDGE_CURVE('',#5631,#5630,#3131,.T.);
#6930=EDGE_CURVE('',#5632,#5631,#3132,.T.);
#6931=EDGE_CURVE('',#5633,#5632,#3133,.T.);
#6932=EDGE_CURVE('',#5634,#5633,#3134,.T.);
#6933=EDGE_CURVE('',#5635,#5634,#3135,.T.);
#6934=EDGE_CURVE('',#5636,#5635,#3136,.T.);
#6935=EDGE_CURVE('',#5616,#5636,#3137,.T.);
#6936=EDGE_CURVE('',#5637,#5617,#3138,.T.);
#6937=EDGE_CURVE('',#5638,#5637,#3139,.T.);
#6938=EDGE_CURVE('',#5639,#5638,#3140,.T.);
#6939=EDGE_CURVE('',#5640,#5639,#3141,.T.);
#6940=EDGE_CURVE('',#5641,#5640,#3142,.T.);
#6941=EDGE_CURVE('',#5642,#5641,#3143,.T.);
#6942=EDGE_CURVE('',#5643,#5642,#3144,.T.);
#6943=EDGE_CURVE('',#5615,#5643,#3145,.T.);
#6944=EDGE_CURVE('',#5644,#5614,#3146,.T.);
#6945=EDGE_CURVE('',#5645,#5644,#3147,.T.);
#6946=EDGE_CURVE('',#5646,#5645,#3148,.T.);
#6947=EDGE_CURVE('',#5647,#5646,#3149,.T.);
#6948=EDGE_CURVE('',#5648,#5647,#3150,.T.);
#6949=EDGE_CURVE('',#5649,#5648,#3151,.T.);
#6950=EDGE_CURVE('',#5650,#5649,#3152,.T.);
#6951=EDGE_CURVE('',#5618,#5650,#3153,.T.);
#6952=EDGE_CURVE('',#5651,#5619,#3154,.T.);
#6953=EDGE_CURVE('',#5652,#5651,#3155,.T.);
#6954=EDGE_CURVE('',#5653,#5652,#3156,.T.);
#6955=EDGE_CURVE('',#5654,#5653,#3157,.T.);
#6956=EDGE_CURVE('',#5655,#5654,#3158,.T.);
#6957=EDGE_CURVE('',#5656,#5655,#3159,.T.);
#6958=EDGE_CURVE('',#5657,#5656,#3160,.T.);
#6959=EDGE_CURVE('',#5613,#5657,#3161,.T.);
#6960=EDGE_CURVE('',#5658,#5612,#3162,.T.);
#6961=EDGE_CURVE('',#5659,#5658,#3163,.T.);
#6962=EDGE_CURVE('',#5660,#5659,#3164,.T.);
#6963=EDGE_CURVE('',#5661,#5660,#3165,.T.);
#6964=EDGE_CURVE('',#5662,#5661,#3166,.T.);
#6965=EDGE_CURVE('',#5663,#5662,#3167,.T.);
#6966=EDGE_CURVE('',#5622,#5663,#3168,.T.);
#6967=EDGE_CURVE('',#5629,#5664,#3169,.T.);
#6968=EDGE_CURVE('',#5665,#5664,#3170,.T.);
#6969=EDGE_CURVE('',#5666,#5665,#3171,.T.);
#6970=EDGE_CURVE('',#5667,#5666,#3172,.T.);
#6971=EDGE_CURVE('',#5667,#5602,#3173,.T.);
#6972=EDGE_CURVE('',#5628,#5668,#3174,.T.);
#6973=EDGE_CURVE('',#5664,#5668,#3175,.T.);
#6974=EDGE_CURVE('',#5669,#5667,#3176,.T.);
#6975=EDGE_CURVE('',#5669,#5603,#3177,.T.);
#6976=EDGE_CURVE('',#5627,#5670,#3178,.T.);
#6977=EDGE_CURVE('',#5668,#5670,#3179,.T.);
#6978=EDGE_CURVE('',#5626,#5671,#3180,.T.);
#6979=EDGE_CURVE('',#5670,#5671,#3181,.T.);
#6980=EDGE_CURVE('',#5625,#5672,#3182,.T.);
#6981=EDGE_CURVE('',#5671,#5672,#3183,.T.);
#6982=EDGE_CURVE('',#5624,#5673,#3184,.T.);
#6983=EDGE_CURVE('',#5672,#5673,#3185,.T.);
#6984=EDGE_CURVE('',#5674,#5623,#3186,.T.);
#6985=EDGE_CURVE('',#5673,#5674,#3187,.T.);
#6986=EDGE_CURVE('',#5675,#5676,#3188,.T.);
#6987=EDGE_CURVE('',#5676,#5677,#3189,.T.);
#6988=EDGE_CURVE('',#5677,#5678,#3190,.T.);
#6989=EDGE_CURVE('',#5678,#5679,#3191,.T.);
#6990=EDGE_CURVE('',#5679,#5680,#3192,.T.);
#6991=EDGE_CURVE('',#5680,#5669,#3193,.T.);
#6992=EDGE_CURVE('',#5666,#5681,#3194,.T.);
#6993=EDGE_CURVE('',#5681,#5682,#3195,.T.);
#6994=EDGE_CURVE('',#5682,#5683,#3196,.T.);
#6995=EDGE_CURVE('',#5683,#5684,#3197,.T.);
#6996=EDGE_CURVE('',#5684,#5685,#3198,.T.);
#6997=EDGE_CURVE('',#5685,#5675,#3199,.T.);
#6998=EDGE_CURVE('',#5677,#5607,#3200,.T.);
#6999=EDGE_CURVE('',#5608,#5676,#3201,.T.);
#7000=EDGE_CURVE('',#5678,#5606,#3202,.T.);
#7001=EDGE_CURVE('',#5679,#5605,#3203,.T.);
#7002=EDGE_CURVE('',#5680,#5604,#3204,.T.);
#7003=EDGE_CURVE('',#5686,#5665,#3205,.T.);
#7004=EDGE_CURVE('',#5681,#5686,#3206,.T.);
#7005=EDGE_CURVE('',#5687,#5686,#3207,.T.);
#7006=EDGE_CURVE('',#5682,#5687,#3208,.T.);
#7007=EDGE_CURVE('',#5688,#5687,#3209,.T.);
#7008=EDGE_CURVE('',#5683,#5688,#3210,.T.);
#7009=EDGE_CURVE('',#5689,#5688,#3211,.T.);
#7010=EDGE_CURVE('',#5684,#5689,#3212,.T.);
#7011=EDGE_CURVE('',#5690,#5689,#3213,.T.);
#7012=EDGE_CURVE('',#5685,#5690,#3214,.T.);
#7013=EDGE_CURVE('',#5691,#5690,#3215,.T.);
#7014=EDGE_CURVE('',#5675,#5691,#3216,.T.);
#7015=EDGE_CURVE('',#5674,#5691,#3217,.T.);
#7016=EDGE_CURVE('',#5657,#5692,#3218,.T.);
#7017=EDGE_CURVE('',#5693,#5692,#3219,.T.);
#7018=EDGE_CURVE('',#5694,#5693,#3220,.T.);
#7019=EDGE_CURVE('',#5695,#5694,#3221,.T.);
#7020=EDGE_CURVE('',#5695,#5566,#3222,.T.);
#7021=EDGE_CURVE('',#5656,#5696,#3223,.T.);
#7022=EDGE_CURVE('',#5692,#5696,#3224,.T.);
#7023=EDGE_CURVE('',#5697,#5695,#3225,.T.);
#7024=EDGE_CURVE('',#5697,#5567,#3226,.T.);
#7025=EDGE_CURVE('',#5655,#5698,#3227,.T.);
#7026=EDGE_CURVE('',#5696,#5698,#3228,.T.);
#7027=EDGE_CURVE('',#5654,#5699,#3229,.T.);
#7028=EDGE_CURVE('',#5698,#5699,#3230,.T.);
#7029=EDGE_CURVE('',#5653,#5700,#3231,.T.);
#7030=EDGE_CURVE('',#5699,#5700,#3232,.T.);
#7031=EDGE_CURVE('',#5652,#5701,#3233,.T.);
#7032=EDGE_CURVE('',#5700,#5701,#3234,.T.);
#7033=EDGE_CURVE('',#5702,#5651,#3235,.T.);
#7034=EDGE_CURVE('',#5701,#5702,#3236,.T.);
#7035=EDGE_CURVE('',#5703,#5704,#3237,.T.);
#7036=EDGE_CURVE('',#5704,#5705,#3238,.T.);
#7037=EDGE_CURVE('',#5705,#5706,#3239,.T.);
#7038=EDGE_CURVE('',#5706,#5707,#3240,.T.);
#7039=EDGE_CURVE('',#5707,#5708,#3241,.T.);
#7040=EDGE_CURVE('',#5708,#5697,#3242,.T.);
#7041=EDGE_CURVE('',#5694,#5709,#3243,.T.);
#7042=EDGE_CURVE('',#5709,#5710,#3244,.T.);
#7043=EDGE_CURVE('',#5710,#5711,#3245,.T.);
#7044=EDGE_CURVE('',#5711,#5712,#3246,.T.);
#7045=EDGE_CURVE('',#5712,#5713,#3247,.T.);
#7046=EDGE_CURVE('',#5713,#5703,#3248,.T.);
#7047=EDGE_CURVE('',#5705,#5571,#3249,.T.);
#7048=EDGE_CURVE('',#5572,#5704,#3250,.T.);
#7049=EDGE_CURVE('',#5706,#5570,#3251,.T.);
#7050=EDGE_CURVE('',#5707,#5569,#3252,.T.);
#7051=EDGE_CURVE('',#5708,#5568,#3253,.T.);
#7052=EDGE_CURVE('',#5714,#5693,#3254,.T.);
#7053=EDGE_CURVE('',#5709,#5714,#3255,.T.);
#7054=EDGE_CURVE('',#5715,#5714,#3256,.T.);
#7055=EDGE_CURVE('',#5710,#5715,#3257,.T.);
#7056=EDGE_CURVE('',#5716,#5715,#3258,.T.);
#7057=EDGE_CURVE('',#5711,#5716,#3259,.T.);
#7058=EDGE_CURVE('',#5717,#5716,#3260,.T.);
#7059=EDGE_CURVE('',#5712,#5717,#3261,.T.);
#7060=EDGE_CURVE('',#5718,#5717,#3262,.T.);
#7061=EDGE_CURVE('',#5713,#5718,#3263,.T.);
#7062=EDGE_CURVE('',#5719,#5718,#3264,.T.);
#7063=EDGE_CURVE('',#5703,#5719,#3265,.T.);
#7064=EDGE_CURVE('',#5702,#5719,#3266,.T.);
#7065=EDGE_CURVE('',#5643,#5720,#3267,.T.);
#7066=EDGE_CURVE('',#5721,#5720,#3268,.T.);
#7067=EDGE_CURVE('',#5722,#5721,#3269,.T.);
#7068=EDGE_CURVE('',#5723,#5722,#3270,.T.);
#7069=EDGE_CURVE('',#5723,#5584,#3271,.T.);
#7070=EDGE_CURVE('',#5642,#5724,#3272,.T.);
#7071=EDGE_CURVE('',#5720,#5724,#3273,.T.);
#7072=EDGE_CURVE('',#5725,#5723,#3274,.T.);
#7073=EDGE_CURVE('',#5725,#5585,#3275,.T.);
#7074=EDGE_CURVE('',#5641,#5726,#3276,.T.);
#7075=EDGE_CURVE('',#5724,#5726,#3277,.T.);
#7076=EDGE_CURVE('',#5640,#5727,#3278,.T.);
#7077=EDGE_CURVE('',#5726,#5727,#3279,.T.);
#7078=EDGE_CURVE('',#5639,#5728,#3280,.T.);
#7079=EDGE_CURVE('',#5727,#5728,#3281,.T.);
#7080=EDGE_CURVE('',#5638,#5729,#3282,.T.);
#7081=EDGE_CURVE('',#5728,#5729,#3283,.T.);
#7082=EDGE_CURVE('',#5730,#5637,#3284,.T.);
#7083=EDGE_CURVE('',#5729,#5730,#3285,.T.);
#7084=EDGE_CURVE('',#5731,#5732,#3286,.T.);
#7085=EDGE_CURVE('',#5732,#5733,#3287,.T.);
#7086=EDGE_CURVE('',#5733,#5734,#3288,.T.);
#7087=EDGE_CURVE('',#5734,#5735,#3289,.T.);
#7088=EDGE_CURVE('',#5735,#5736,#3290,.T.);
#7089=EDGE_CURVE('',#5736,#5725,#3291,.T.);
#7090=EDGE_CURVE('',#5722,#5737,#3292,.T.);
#7091=EDGE_CURVE('',#5737,#5738,#3293,.T.);
#7092=EDGE_CURVE('',#5738,#5739,#3294,.T.);
#7093=EDGE_CURVE('',#5739,#5740,#3295,.T.);
#7094=EDGE_CURVE('',#5740,#5741,#3296,.T.);
#7095=EDGE_CURVE('',#5741,#5731,#3297,.T.);
#7096=EDGE_CURVE('',#5733,#5589,#3298,.T.);
#7097=EDGE_CURVE('',#5590,#5732,#3299,.T.);
#7098=EDGE_CURVE('',#5734,#5588,#3300,.T.);
#7099=EDGE_CURVE('',#5735,#5587,#3301,.T.);
#7100=EDGE_CURVE('',#5736,#5586,#3302,.T.);
#7101=EDGE_CURVE('',#5742,#5721,#3303,.T.);
#7102=EDGE_CURVE('',#5737,#5742,#3304,.T.);
#7103=EDGE_CURVE('',#5743,#5742,#3305,.T.);
#7104=EDGE_CURVE('',#5738,#5743,#3306,.T.);
#7105=EDGE_CURVE('',#5744,#5743,#3307,.T.);
#7106=EDGE_CURVE('',#5739,#5744,#3308,.T.);
#7107=EDGE_CURVE('',#5745,#5744,#3309,.T.);
#7108=EDGE_CURVE('',#5740,#5745,#3310,.T.);
#7109=EDGE_CURVE('',#5746,#5745,#3311,.T.);
#7110=EDGE_CURVE('',#5741,#5746,#3312,.T.);
#7111=EDGE_CURVE('',#5747,#5746,#3313,.T.);
#7112=EDGE_CURVE('',#5731,#5747,#3314,.T.);
#7113=EDGE_CURVE('',#5730,#5747,#3315,.T.);
#7114=EDGE_CURVE('',#5636,#5748,#3316,.T.);
#7115=EDGE_CURVE('',#5749,#5748,#3317,.T.);
#7116=EDGE_CURVE('',#5750,#5749,#3318,.T.);
#7117=EDGE_CURVE('',#5751,#5750,#3319,.T.);
#7118=EDGE_CURVE('',#5751,#5593,#3320,.T.);
#7119=EDGE_CURVE('',#5635,#5752,#3321,.T.);
#7120=EDGE_CURVE('',#5748,#5752,#3322,.T.);
#7121=EDGE_CURVE('',#5753,#5751,#3323,.T.);
#7122=EDGE_CURVE('',#5753,#5594,#3324,.T.);
#7123=EDGE_CURVE('',#5634,#5754,#3325,.T.);
#7124=EDGE_CURVE('',#5752,#5754,#3326,.T.);
#7125=EDGE_CURVE('',#5633,#5755,#3327,.T.);
#7126=EDGE_CURVE('',#5754,#5755,#3328,.T.);
#7127=EDGE_CURVE('',#5632,#5756,#3329,.T.);
#7128=EDGE_CURVE('',#5755,#5756,#3330,.T.);
#7129=EDGE_CURVE('',#5631,#5757,#3331,.T.);
#7130=EDGE_CURVE('',#5756,#5757,#3332,.T.);
#7131=EDGE_CURVE('',#5758,#5630,#3333,.T.);
#7132=EDGE_CURVE('',#5757,#5758,#3334,.T.);
#7133=EDGE_CURVE('',#5759,#5760,#3335,.T.);
#7134=EDGE_CURVE('',#5760,#5761,#3336,.T.);
#7135=EDGE_CURVE('',#5761,#5762,#3337,.T.);
#7136=EDGE_CURVE('',#5762,#5763,#3338,.T.);
#7137=EDGE_CURVE('',#5763,#5764,#3339,.T.);
#7138=EDGE_CURVE('',#5764,#5753,#3340,.T.);
#7139=EDGE_CURVE('',#5750,#5765,#3341,.T.);
#7140=EDGE_CURVE('',#5765,#5766,#3342,.T.);
#7141=EDGE_CURVE('',#5766,#5767,#3343,.T.);
#7142=EDGE_CURVE('',#5767,#5768,#3344,.T.);
#7143=EDGE_CURVE('',#5768,#5769,#3345,.T.);
#7144=EDGE_CURVE('',#5769,#5759,#3346,.T.);
#7145=EDGE_CURVE('',#5761,#5598,#3347,.T.);
#7146=EDGE_CURVE('',#5599,#5760,#3348,.T.);
#7147=EDGE_CURVE('',#5762,#5597,#3349,.T.);
#7148=EDGE_CURVE('',#5763,#5596,#3350,.T.);
#7149=EDGE_CURVE('',#5764,#5595,#3351,.T.);
#7150=EDGE_CURVE('',#5770,#5749,#3352,.T.);
#7151=EDGE_CURVE('',#5765,#5770,#3353,.T.);
#7152=EDGE_CURVE('',#5771,#5770,#3354,.T.);
#7153=EDGE_CURVE('',#5766,#5771,#3355,.T.);
#7154=EDGE_CURVE('',#5772,#5771,#3356,.T.);
#7155=EDGE_CURVE('',#5767,#5772,#3357,.T.);
#7156=EDGE_CURVE('',#5773,#5772,#3358,.T.);
#7157=EDGE_CURVE('',#5768,#5773,#3359,.T.);
#7158=EDGE_CURVE('',#5774,#5773,#3360,.T.);
#7159=EDGE_CURVE('',#5769,#5774,#3361,.T.);
#7160=EDGE_CURVE('',#5775,#5774,#3362,.T.);
#7161=EDGE_CURVE('',#5759,#5775,#3363,.T.);
#7162=EDGE_CURVE('',#5758,#5775,#3364,.T.);
#7163=EDGE_CURVE('',#5650,#5776,#3365,.T.);
#7164=EDGE_CURVE('',#5777,#5776,#3366,.T.);
#7165=EDGE_CURVE('',#5778,#5777,#3367,.T.);
#7166=EDGE_CURVE('',#5779,#5778,#3368,.T.);
#7167=EDGE_CURVE('',#5779,#5575,#3369,.T.);
#7168=EDGE_CURVE('',#5649,#5780,#3370,.T.);
#7169=EDGE_CURVE('',#5776,#5780,#3371,.T.);
#7170=EDGE_CURVE('',#5781,#5779,#3372,.T.);
#7171=EDGE_CURVE('',#5781,#5576,#3373,.T.);
#7172=EDGE_CURVE('',#5648,#5782,#3374,.T.);
#7173=EDGE_CURVE('',#5780,#5782,#3375,.T.);
#7174=EDGE_CURVE('',#5647,#5783,#3376,.T.);
#7175=EDGE_CURVE('',#5782,#5783,#3377,.T.);
#7176=EDGE_CURVE('',#5646,#5784,#3378,.T.);
#7177=EDGE_CURVE('',#5783,#5784,#3379,.T.);
#7178=EDGE_CURVE('',#5645,#5785,#3380,.T.);
#7179=EDGE_CURVE('',#5784,#5785,#3381,.T.);
#7180=EDGE_CURVE('',#5786,#5644,#3382,.T.);
#7181=EDGE_CURVE('',#5785,#5786,#3383,.T.);
#7182=EDGE_CURVE('',#5787,#5788,#3384,.T.);
#7183=EDGE_CURVE('',#5788,#5789,#3385,.T.);
#7184=EDGE_CURVE('',#5789,#5790,#3386,.T.);
#7185=EDGE_CURVE('',#5790,#5791,#3387,.T.);
#7186=EDGE_CURVE('',#5791,#5792,#3388,.T.);
#7187=EDGE_CURVE('',#5792,#5781,#3389,.T.);
#7188=EDGE_CURVE('',#5778,#5793,#3390,.T.);
#7189=EDGE_CURVE('',#5793,#5794,#3391,.T.);
#7190=EDGE_CURVE('',#5794,#5795,#3392,.T.);
#7191=EDGE_CURVE('',#5795,#5796,#3393,.T.);
#7192=EDGE_CURVE('',#5796,#5797,#3394,.T.);
#7193=EDGE_CURVE('',#5797,#5787,#3395,.T.);
#7194=EDGE_CURVE('',#5789,#5580,#3396,.T.);
#7195=EDGE_CURVE('',#5581,#5788,#3397,.T.);
#7196=EDGE_CURVE('',#5790,#5579,#3398,.T.);
#7197=EDGE_CURVE('',#5791,#5578,#3399,.T.);
#7198=EDGE_CURVE('',#5792,#5577,#3400,.T.);
#7199=EDGE_CURVE('',#5798,#5777,#3401,.T.);
#7200=EDGE_CURVE('',#5793,#5798,#3402,.T.);
#7201=EDGE_CURVE('',#5799,#5798,#3403,.T.);
#7202=EDGE_CURVE('',#5794,#5799,#3404,.T.);
#7203=EDGE_CURVE('',#5800,#5799,#3405,.T.);
#7204=EDGE_CURVE('',#5795,#5800,#3406,.T.);
#7205=EDGE_CURVE('',#5801,#5800,#3407,.T.);
#7206=EDGE_CURVE('',#5796,#5801,#3408,.T.);
#7207=EDGE_CURVE('',#5802,#5801,#3409,.T.);
#7208=EDGE_CURVE('',#5797,#5802,#3410,.T.);
#7209=EDGE_CURVE('',#5803,#5802,#3411,.T.);
#7210=EDGE_CURVE('',#5787,#5803,#3412,.T.);
#7211=EDGE_CURVE('',#5786,#5803,#3413,.T.);
#7212=EDGE_CURVE('',#5622,#5804,#3414,.T.);
#7213=EDGE_CURVE('',#5805,#5804,#3415,.T.);
#7214=EDGE_CURVE('',#5806,#5805,#3416,.T.);
#7215=EDGE_CURVE('',#5807,#5806,#3417,.T.);
#7216=EDGE_CURVE('',#5807,#5556,#3418,.T.);
#7217=EDGE_CURVE('',#5663,#5808,#3419,.T.);
#7218=EDGE_CURVE('',#5804,#5808,#3420,.T.);
#7219=EDGE_CURVE('',#5809,#5807,#3421,.T.);
#7220=EDGE_CURVE('',#5809,#5558,#3422,.T.);
#7221=EDGE_CURVE('',#5662,#5810,#3423,.T.);
#7222=EDGE_CURVE('',#5808,#5810,#3424,.T.);
#7223=EDGE_CURVE('',#5661,#5811,#3425,.T.);
#7224=EDGE_CURVE('',#5810,#5811,#3426,.T.);
#7225=EDGE_CURVE('',#5660,#5812,#3427,.T.);
#7226=EDGE_CURVE('',#5811,#5812,#3428,.T.);
#7227=EDGE_CURVE('',#5659,#5813,#3429,.T.);
#7228=EDGE_CURVE('',#5812,#5813,#3430,.T.);
#7229=EDGE_CURVE('',#5814,#5658,#3431,.T.);
#7230=EDGE_CURVE('',#5813,#5814,#3432,.T.);
#7231=EDGE_CURVE('',#5815,#5816,#3433,.T.);
#7232=EDGE_CURVE('',#5816,#5817,#3434,.T.);
#7233=EDGE_CURVE('',#5817,#5818,#3435,.T.);
#7234=EDGE_CURVE('',#5818,#5819,#3436,.T.);
#7235=EDGE_CURVE('',#5819,#5820,#3437,.T.);
#7236=EDGE_CURVE('',#5820,#5809,#3438,.T.);
#7237=EDGE_CURVE('',#5806,#5821,#3439,.T.);
#7238=EDGE_CURVE('',#5821,#5822,#3440,.T.);
#7239=EDGE_CURVE('',#5822,#5823,#3441,.T.);
#7240=EDGE_CURVE('',#5823,#5824,#3442,.T.);
#7241=EDGE_CURVE('',#5824,#5825,#3443,.T.);
#7242=EDGE_CURVE('',#5825,#5815,#3444,.T.);
#7243=EDGE_CURVE('',#5817,#5562,#3445,.T.);
#7244=EDGE_CURVE('',#5563,#5816,#3446,.T.);
#7245=EDGE_CURVE('',#5818,#5561,#3447,.T.);
#7246=EDGE_CURVE('',#5819,#5560,#3448,.T.);
#7247=EDGE_CURVE('',#5820,#5559,#3449,.T.);
#7248=EDGE_CURVE('',#5826,#5805,#3450,.T.);
#7249=EDGE_CURVE('',#5821,#5826,#3451,.T.);
#7250=EDGE_CURVE('',#5827,#5826,#3452,.T.);
#7251=EDGE_CURVE('',#5822,#5827,#3453,.T.);
#7252=EDGE_CURVE('',#5828,#5827,#3454,.T.);
#7253=EDGE_CURVE('',#5823,#5828,#3455,.T.);
#7254=EDGE_CURVE('',#5829,#5828,#3456,.T.);
#7255=EDGE_CURVE('',#5824,#5829,#3457,.T.);
#7256=EDGE_CURVE('',#5830,#5829,#3458,.T.);
#7257=EDGE_CURVE('',#5825,#5830,#3459,.T.);
#7258=EDGE_CURVE('',#5831,#5830,#3460,.T.);
#7259=EDGE_CURVE('',#5815,#5831,#3461,.T.);
#7260=EDGE_CURVE('',#5814,#5831,#3462,.T.);
#9272=ORIENTED_EDGE('',*,*,#6847,.F.);
#9273=ORIENTED_EDGE('',*,*,#6848,.F.);
#9274=ORIENTED_EDGE('',*,*,#6849,.F.);
#9275=ORIENTED_EDGE('',*,*,#6850,.F.);
#9276=ORIENTED_EDGE('',*,*,#6851,.F.);
#9277=ORIENTED_EDGE('',*,*,#6852,.F.);
#9278=ORIENTED_EDGE('',*,*,#6853,.F.);
#9279=ORIENTED_EDGE('',*,*,#6854,.F.);
#9280=ORIENTED_EDGE('',*,*,#6855,.T.);
#9281=ORIENTED_EDGE('',*,*,#6856,.F.);
#9282=ORIENTED_EDGE('',*,*,#6857,.F.);
#9283=ORIENTED_EDGE('',*,*,#6858,.F.);
#9284=ORIENTED_EDGE('',*,*,#6859,.F.);
#9285=ORIENTED_EDGE('',*,*,#6860,.F.);
#9286=ORIENTED_EDGE('',*,*,#6861,.F.);
#9287=ORIENTED_EDGE('',*,*,#6862,.F.);
#9288=ORIENTED_EDGE('',*,*,#6863,.F.);
#9289=ORIENTED_EDGE('',*,*,#6864,.T.);
#9290=ORIENTED_EDGE('',*,*,#6865,.F.);
#9291=ORIENTED_EDGE('',*,*,#6866,.F.);
#9292=ORIENTED_EDGE('',*,*,#6867,.F.);
#9293=ORIENTED_EDGE('',*,*,#6868,.F.);
#9294=ORIENTED_EDGE('',*,*,#6869,.F.);
#9295=ORIENTED_EDGE('',*,*,#6870,.F.);
#9296=ORIENTED_EDGE('',*,*,#6871,.F.);
#9297=ORIENTED_EDGE('',*,*,#6872,.F.);
#9298=ORIENTED_EDGE('',*,*,#6873,.T.);
#9299=ORIENTED_EDGE('',*,*,#6874,.F.);
#9300=ORIENTED_EDGE('',*,*,#6875,.F.);
#9301=ORIENTED_EDGE('',*,*,#6876,.F.);
#9302=ORIENTED_EDGE('',*,*,#6877,.F.);
#9303=ORIENTED_EDGE('',*,*,#6878,.F.);
#9304=ORIENTED_EDGE('',*,*,#6879,.F.);
#9305=ORIENTED_EDGE('',*,*,#6880,.F.);
#9306=ORIENTED_EDGE('',*,*,#6881,.F.);
#9307=ORIENTED_EDGE('',*,*,#6882,.T.);
#9308=ORIENTED_EDGE('',*,*,#6883,.F.);
#9309=ORIENTED_EDGE('',*,*,#6884,.F.);
#9310=ORIENTED_EDGE('',*,*,#6885,.F.);
#9311=ORIENTED_EDGE('',*,*,#6886,.F.);
#9312=ORIENTED_EDGE('',*,*,#6887,.F.);
#9313=ORIENTED_EDGE('',*,*,#6888,.F.);
#9314=ORIENTED_EDGE('',*,*,#6889,.F.);
#9315=ORIENTED_EDGE('',*,*,#6890,.F.);
#9316=ORIENTED_EDGE('',*,*,#6891,.T.);
#9317=ORIENTED_EDGE('',*,*,#6892,.F.);
#9318=ORIENTED_EDGE('',*,*,#6893,.F.);
#9319=ORIENTED_EDGE('',*,*,#6894,.F.);
#9320=ORIENTED_EDGE('',*,*,#6895,.F.);
#9321=ORIENTED_EDGE('',*,*,#6896,.F.);
#9322=ORIENTED_EDGE('',*,*,#6897,.F.);
#9323=ORIENTED_EDGE('',*,*,#6898,.F.);
#9324=ORIENTED_EDGE('',*,*,#6899,.F.);
#9325=ORIENTED_EDGE('',*,*,#6900,.T.);
#9326=ORIENTED_EDGE('',*,*,#6901,.F.);
#9327=ORIENTED_EDGE('',*,*,#6902,.F.);
#9328=ORIENTED_EDGE('',*,*,#6903,.F.);
#9329=ORIENTED_EDGE('',*,*,#6891,.F.);
#9330=ORIENTED_EDGE('',*,*,#6904,.F.);
#9331=ORIENTED_EDGE('',*,*,#6905,.F.);
#9332=ORIENTED_EDGE('',*,*,#6906,.F.);
#9333=ORIENTED_EDGE('',*,*,#6855,.F.);
#9334=ORIENTED_EDGE('',*,*,#6907,.F.);
#9335=ORIENTED_EDGE('',*,*,#6908,.F.);
#9336=ORIENTED_EDGE('',*,*,#6909,.F.);
#9337=ORIENTED_EDGE('',*,*,#6873,.F.);
#9338=ORIENTED_EDGE('',*,*,#6910,.F.);
#9339=ORIENTED_EDGE('',*,*,#6882,.F.);
#9340=ORIENTED_EDGE('',*,*,#6911,.F.);
#9341=ORIENTED_EDGE('',*,*,#6912,.F.);
#9342=ORIENTED_EDGE('',*,*,#6913,.F.);
#9343=ORIENTED_EDGE('',*,*,#6864,.F.);
#9344=ORIENTED_EDGE('',*,*,#6914,.F.);
#9345=ORIENTED_EDGE('',*,*,#6915,.F.);
#9346=ORIENTED_EDGE('',*,*,#6916,.F.);
#9347=ORIENTED_EDGE('',*,*,#6900,.F.);
#9348=ORIENTED_EDGE('',*,*,#6917,.F.);
#9349=ORIENTED_EDGE('',*,*,#6918,.F.);
#9350=ORIENTED_EDGE('',*,*,#6919,.F.);
#9351=ORIENTED_EDGE('',*,*,#6918,.T.);
#9352=ORIENTED_EDGE('',*,*,#6920,.F.);
#9353=ORIENTED_EDGE('',*,*,#6921,.F.);
#9354=ORIENTED_EDGE('',*,*,#6922,.F.);
#9355=ORIENTED_EDGE('',*,*,#6923,.F.);
#9356=ORIENTED_EDGE('',*,*,#6924,.F.);
#9357=ORIENTED_EDGE('',*,*,#6925,.F.);
#9358=ORIENTED_EDGE('',*,*,#6926,.F.);
#9359=ORIENTED_EDGE('',*,*,#6927,.F.);
#9360=ORIENTED_EDGE('',*,*,#6902,.T.);
#9361=ORIENTED_EDGE('',*,*,#6928,.F.);
#9362=ORIENTED_EDGE('',*,*,#6929,.F.);
#9363=ORIENTED_EDGE('',*,*,#6930,.F.);
#9364=ORIENTED_EDGE('',*,*,#6931,.F.);
#9365=ORIENTED_EDGE('',*,*,#6932,.F.);
#9366=ORIENTED_EDGE('',*,*,#6933,.F.);
#9367=ORIENTED_EDGE('',*,*,#6934,.F.);
#9368=ORIENTED_EDGE('',*,*,#6935,.F.);
#9369=ORIENTED_EDGE('',*,*,#6912,.T.);
#9370=ORIENTED_EDGE('',*,*,#6936,.F.);
#9371=ORIENTED_EDGE('',*,*,#6937,.F.);
#9372=ORIENTED_EDGE('',*,*,#6938,.F.);
#9373=ORIENTED_EDGE('',*,*,#6939,.F.);
#9374=ORIENTED_EDGE('',*,*,#6940,.F.);
#9375=ORIENTED_EDGE('',*,*,#6941,.F.);
#9376=ORIENTED_EDGE('',*,*,#6942,.F.);
#9377=ORIENTED_EDGE('',*,*,#6943,.F.);
#9378=ORIENTED_EDGE('',*,*,#6908,.T.);
#9379=ORIENTED_EDGE('',*,*,#6944,.F.);
#9380=ORIENTED_EDGE('',*,*,#6945,.F.);
#9381=ORIENTED_EDGE('',*,*,#6946,.F.);
#9382=ORIENTED_EDGE('',*,*,#6947,.F.);
#9383=ORIENTED_EDGE('',*,*,#6948,.F.);
#9384=ORIENTED_EDGE('',*,*,#6949,.F.);
#9385=ORIENTED_EDGE('',*,*,#6950,.F.);
#9386=ORIENTED_EDGE('',*,*,#6951,.F.);
#9387=ORIENTED_EDGE('',*,*,#6915,.T.);
#9388=ORIENTED_EDGE('',*,*,#6952,.F.);
#9389=ORIENTED_EDGE('',*,*,#6953,.F.);
#9390=ORIENTED_EDGE('',*,*,#6954,.F.);
#9391=ORIENTED_EDGE('',*,*,#6955,.F.);
#9392=ORIENTED_EDGE('',*,*,#6956,.F.);
#9393=ORIENTED_EDGE('',*,*,#6957,.F.);
#9394=ORIENTED_EDGE('',*,*,#6958,.F.);
#9395=ORIENTED_EDGE('',*,*,#6959,.F.);
#9396=ORIENTED_EDGE('',*,*,#6905,.T.);
#9397=ORIENTED_EDGE('',*,*,#6960,.F.);
#9398=ORIENTED_EDGE('',*,*,#6961,.F.);
#9399=ORIENTED_EDGE('',*,*,#6962,.F.);
#9400=ORIENTED_EDGE('',*,*,#6963,.F.);
#9401=ORIENTED_EDGE('',*,*,#6964,.F.);
#9402=ORIENTED_EDGE('',*,*,#6965,.F.);
#9403=ORIENTED_EDGE('',*,*,#6966,.F.);
#9404=ORIENTED_EDGE('',*,*,#6892,.T.);
#9405=ORIENTED_EDGE('',*,*,#6903,.T.);
#9406=ORIENTED_EDGE('',*,*,#6927,.T.);
#9407=ORIENTED_EDGE('',*,*,#6967,.T.);
#9408=ORIENTED_EDGE('',*,*,#6968,.F.);
#9409=ORIENTED_EDGE('',*,*,#6969,.F.);
#9410=ORIENTED_EDGE('',*,*,#6970,.F.);
#9411=ORIENTED_EDGE('',*,*,#6971,.T.);
#9412=ORIENTED_EDGE('',*,*,#6926,.T.);
#9413=ORIENTED_EDGE('',*,*,#6972,.T.);
#9414=ORIENTED_EDGE('',*,*,#6973,.F.);
#9415=ORIENTED_EDGE('',*,*,#6967,.F.);
#9416=ORIENTED_EDGE('',*,*,#6893,.T.);
#9417=ORIENTED_EDGE('',*,*,#6971,.F.);
#9418=ORIENTED_EDGE('',*,*,#6974,.F.);
#9419=ORIENTED_EDGE('',*,*,#6975,.T.);
#9420=ORIENTED_EDGE('',*,*,#6925,.T.);
#9421=ORIENTED_EDGE('',*,*,#6976,.T.);
#9422=ORIENTED_EDGE('',*,*,#6977,.F.);
#9423=ORIENTED_EDGE('',*,*,#6972,.F.);
#9424=ORIENTED_EDGE('',*,*,#6924,.T.);
#9425=ORIENTED_EDGE('',*,*,#6978,.T.);
#9426=ORIENTED_EDGE('',*,*,#6979,.F.);
#9427=ORIENTED_EDGE('',*,*,#6976,.F.);
#9428=ORIENTED_EDGE('',*,*,#6923,.T.);
#9429=ORIENTED_EDGE('',*,*,#6980,.T.);
#9430=ORIENTED_EDGE('',*,*,#6981,.F.);
#9431=ORIENTED_EDGE('',*,*,#6978,.F.);
#9432=ORIENTED_EDGE('',*,*,#6922,.T.);
#9433=ORIENTED_EDGE('',*,*,#6982,.T.);
#9434=ORIENTED_EDGE('',*,*,#6983,.F.);
#9435=ORIENTED_EDGE('',*,*,#6980,.F.);
#9436=ORIENTED_EDGE('',*,*,#6921,.T.);
#9437=ORIENTED_EDGE('',*,*,#6984,.F.);
#9438=ORIENTED_EDGE('',*,*,#6985,.F.);
#9439=ORIENTED_EDGE('',*,*,#6982,.F.);
#9440=ORIENTED_EDGE('',*,*,#6986,.T.);
#9441=ORIENTED_EDGE('',*,*,#6987,.T.);
#9442=ORIENTED_EDGE('',*,*,#6988,.T.);
#9443=ORIENTED_EDGE('',*,*,#6989,.T.);
#9444=ORIENTED_EDGE('',*,*,#6990,.T.);
#9445=ORIENTED_EDGE('',*,*,#6991,.T.);
#9446=ORIENTED_EDGE('',*,*,#6974,.T.);
#9447=ORIENTED_EDGE('',*,*,#6970,.T.);
#9448=ORIENTED_EDGE('',*,*,#6992,.T.);
#9449=ORIENTED_EDGE('',*,*,#6993,.T.);
#9450=ORIENTED_EDGE('',*,*,#6994,.T.);
#9451=ORIENTED_EDGE('',*,*,#6995,.T.);
#9452=ORIENTED_EDGE('',*,*,#6996,.T.);
#9453=ORIENTED_EDGE('',*,*,#6997,.T.);
#9454=ORIENTED_EDGE('',*,*,#6898,.T.);
#9455=ORIENTED_EDGE('',*,*,#6998,.F.);
#9456=ORIENTED_EDGE('',*,*,#6987,.F.);
#9457=ORIENTED_EDGE('',*,*,#6999,.F.);
#9458=ORIENTED_EDGE('',*,*,#6897,.T.);
#9459=ORIENTED_EDGE('',*,*,#7000,.F.);
#9460=ORIENTED_EDGE('',*,*,#6988,.F.);
#9461=ORIENTED_EDGE('',*,*,#6998,.T.);
#9462=ORIENTED_EDGE('',*,*,#6896,.T.);
#9463=ORIENTED_EDGE('',*,*,#7001,.F.);
#9464=ORIENTED_EDGE('',*,*,#6989,.F.);
#9465=ORIENTED_EDGE('',*,*,#7000,.T.);
#9466=ORIENTED_EDGE('',*,*,#6895,.T.);
#9467=ORIENTED_EDGE('',*,*,#7002,.F.);
#9468=ORIENTED_EDGE('',*,*,#6990,.F.);
#9469=ORIENTED_EDGE('',*,*,#7001,.T.);
#9470=ORIENTED_EDGE('',*,*,#6894,.T.);
#9471=ORIENTED_EDGE('',*,*,#6975,.F.);
#9472=ORIENTED_EDGE('',*,*,#6991,.F.);
#9473=ORIENTED_EDGE('',*,*,#7002,.T.);
#9474=ORIENTED_EDGE('',*,*,#6969,.T.);
#9475=ORIENTED_EDGE('',*,*,#7003,.F.);
#9476=ORIENTED_EDGE('',*,*,#7004,.F.);
#9477=ORIENTED_EDGE('',*,*,#6992,.F.);
#9478=ORIENTED_EDGE('',*,*,#7004,.T.);
#9479=ORIENTED_EDGE('',*,*,#7005,.F.);
#9480=ORIENTED_EDGE('',*,*,#7006,.F.);
#9481=ORIENTED_EDGE('',*,*,#6993,.F.);
#9482=ORIENTED_EDGE('',*,*,#7006,.T.);
#9483=ORIENTED_EDGE('',*,*,#7007,.F.);
#9484=ORIENTED_EDGE('',*,*,#7008,.F.);
#9485=ORIENTED_EDGE('',*,*,#6994,.F.);
#9486=ORIENTED_EDGE('',*,*,#7008,.T.);
#9487=ORIENTED_EDGE('',*,*,#7009,.F.);
#9488=ORIENTED_EDGE('',*,*,#7010,.F.);
#9489=ORIENTED_EDGE('',*,*,#6995,.F.);
#9490=ORIENTED_EDGE('',*,*,#7010,.T.);
#9491=ORIENTED_EDGE('',*,*,#7011,.F.);
#9492=ORIENTED_EDGE('',*,*,#7012,.F.);
#9493=ORIENTED_EDGE('',*,*,#6996,.F.);
#9494=ORIENTED_EDGE('',*,*,#7012,.T.);
#9495=ORIENTED_EDGE('',*,*,#7013,.F.);
#9496=ORIENTED_EDGE('',*,*,#7014,.F.);
#9497=ORIENTED_EDGE('',*,*,#6997,.F.);
#9498=ORIENTED_EDGE('',*,*,#6899,.T.);
#9499=ORIENTED_EDGE('',*,*,#6999,.T.);
#9500=ORIENTED_EDGE('',*,*,#6986,.F.);
#9501=ORIENTED_EDGE('',*,*,#7014,.T.);
#9502=ORIENTED_EDGE('',*,*,#7015,.F.);
#9503=ORIENTED_EDGE('',*,*,#6984,.T.);
#9504=ORIENTED_EDGE('',*,*,#6920,.T.);
#9505=ORIENTED_EDGE('',*,*,#6917,.T.);
#9506=ORIENTED_EDGE('',*,*,#7015,.T.);
#9507=ORIENTED_EDGE('',*,*,#7013,.T.);
#9508=ORIENTED_EDGE('',*,*,#7011,.T.);
#9509=ORIENTED_EDGE('',*,*,#7009,.T.);
#9510=ORIENTED_EDGE('',*,*,#7007,.T.);
#9511=ORIENTED_EDGE('',*,*,#7005,.T.);
#9512=ORIENTED_EDGE('',*,*,#7003,.T.);
#9513=ORIENTED_EDGE('',*,*,#6968,.T.);
#9514=ORIENTED_EDGE('',*,*,#6973,.T.);
#9515=ORIENTED_EDGE('',*,*,#6977,.T.);
#9516=ORIENTED_EDGE('',*,*,#6979,.T.);
#9517=ORIENTED_EDGE('',*,*,#6981,.T.);
#9518=ORIENTED_EDGE('',*,*,#6983,.T.);
#9519=ORIENTED_EDGE('',*,*,#6985,.T.);
#9520=ORIENTED_EDGE('',*,*,#6856,.T.);
#9521=ORIENTED_EDGE('',*,*,#6906,.T.);
#9522=ORIENTED_EDGE('',*,*,#6959,.T.);
#9523=ORIENTED_EDGE('',*,*,#7016,.T.);
#9524=ORIENTED_EDGE('',*,*,#7017,.F.);
#9525=ORIENTED_EDGE('',*,*,#7018,.F.);
#9526=ORIENTED_EDGE('',*,*,#7019,.F.);
#9527=ORIENTED_EDGE('',*,*,#7020,.T.);
#9528=ORIENTED_EDGE('',*,*,#6958,.T.);
#9529=ORIENTED_EDGE('',*,*,#7021,.T.);
#9530=ORIENTED_EDGE('',*,*,#7022,.F.);
#9531=ORIENTED_EDGE('',*,*,#7016,.F.);
#9532=ORIENTED_EDGE('',*,*,#6857,.T.);
#9533=ORIENTED_EDGE('',*,*,#7020,.F.);
#9534=ORIENTED_EDGE('',*,*,#7023,.F.);
#9535=ORIENTED_EDGE('',*,*,#7024,.T.);
#9536=ORIENTED_EDGE('',*,*,#6957,.T.);
#9537=ORIENTED_EDGE('',*,*,#7025,.T.);
#9538=ORIENTED_EDGE('',*,*,#7026,.F.);
#9539=ORIENTED_EDGE('',*,*,#7021,.F.);
#9540=ORIENTED_EDGE('',*,*,#6956,.T.);
#9541=ORIENTED_EDGE('',*,*,#7027,.T.);
#9542=ORIENTED_EDGE('',*,*,#7028,.F.);
#9543=ORIENTED_EDGE('',*,*,#7025,.F.);
#9544=ORIENTED_EDGE('',*,*,#6955,.T.);
#9545=ORIENTED_EDGE('',*,*,#7029,.T.);
#9546=ORIENTED_EDGE('',*,*,#7030,.F.);
#9547=ORIENTED_EDGE('',*,*,#7027,.F.);
#9548=ORIENTED_EDGE('',*,*,#6954,.T.);
#9549=ORIENTED_EDGE('',*,*,#7031,.T.);
#9550=ORIENTED_EDGE('',*,*,#7032,.F.);
#9551=ORIENTED_EDGE('',*,*,#7029,.F.);
#9552=ORIENTED_EDGE('',*,*,#6953,.T.);
#9553=ORIENTED_EDGE('',*,*,#7033,.F.);
#9554=ORIENTED_EDGE('',*,*,#7034,.F.);
#9555=ORIENTED_EDGE('',*,*,#7031,.F.);
#9556=ORIENTED_EDGE('',*,*,#7035,.T.);
#9557=ORIENTED_EDGE('',*,*,#7036,.T.);
#9558=ORIENTED_EDGE('',*,*,#7037,.T.);
#9559=ORIENTED_EDGE('',*,*,#7038,.T.);
#9560=ORIENTED_EDGE('',*,*,#7039,.T.);
#9561=ORIENTED_EDGE('',*,*,#7040,.T.);
#9562=ORIENTED_EDGE('',*,*,#7023,.T.);
#9563=ORIENTED_EDGE('',*,*,#7019,.T.);
#9564=ORIENTED_EDGE('',*,*,#7041,.T.);
#9565=ORIENTED_EDGE('',*,*,#7042,.T.);
#9566=ORIENTED_EDGE('',*,*,#7043,.T.);
#9567=ORIENTED_EDGE('',*,*,#7044,.T.);
#9568=ORIENTED_EDGE('',*,*,#7045,.T.);
#9569=ORIENTED_EDGE('',*,*,#7046,.T.);
#9570=ORIENTED_EDGE('',*,*,#6862,.T.);
#9571=ORIENTED_EDGE('',*,*,#7047,.F.);
#9572=ORIENTED_EDGE('',*,*,#7036,.F.);
#9573=ORIENTED_EDGE('',*,*,#7048,.F.);
#9574=ORIENTED_EDGE('',*,*,#6861,.T.);
#9575=ORIENTED_EDGE('',*,*,#7049,.F.);
#9576=ORIENTED_EDGE('',*,*,#7037,.F.);
#9577=ORIENTED_EDGE('',*,*,#7047,.T.);
#9578=ORIENTED_EDGE('',*,*,#6860,.T.);
#9579=ORIENTED_EDGE('',*,*,#7050,.F.);
#9580=ORIENTED_EDGE('',*,*,#7038,.F.);
#9581=ORIENTED_EDGE('',*,*,#7049,.T.);
#9582=ORIENTED_EDGE('',*,*,#6859,.T.);
#9583=ORIENTED_EDGE('',*,*,#7051,.F.);
#9584=ORIENTED_EDGE('',*,*,#7039,.F.);
#9585=ORIENTED_EDGE('',*,*,#7050,.T.);
#9586=ORIENTED_EDGE('',*,*,#6858,.T.);
#9587=ORIENTED_EDGE('',*,*,#7024,.F.);
#9588=ORIENTED_EDGE('',*,*,#7040,.F.);
#9589=ORIENTED_EDGE('',*,*,#7051,.T.);
#9590=ORIENTED_EDGE('',*,*,#7018,.T.);
#9591=ORIENTED_EDGE('',*,*,#7052,.F.);
#9592=ORIENTED_EDGE('',*,*,#7053,.F.);
#9593=ORIENTED_EDGE('',*,*,#7041,.F.);
#9594=ORIENTED_EDGE('',*,*,#7053,.T.);
#9595=ORIENTED_EDGE('',*,*,#7054,.F.);
#9596=ORIENTED_EDGE('',*,*,#7055,.F.);
#9597=ORIENTED_EDGE('',*,*,#7042,.F.);
#9598=ORIENTED_EDGE('',*,*,#7055,.T.);
#9599=ORIENTED_EDGE('',*,*,#7056,.F.);
#9600=ORIENTED_EDGE('',*,*,#7057,.F.);
#9601=ORIENTED_EDGE('',*,*,#7043,.F.);
#9602=ORIENTED_EDGE('',*,*,#7057,.T.);
#9603=ORIENTED_EDGE('',*,*,#7058,.F.);
#9604=ORIENTED_EDGE('',*,*,#7059,.F.);
#9605=ORIENTED_EDGE('',*,*,#7044,.F.);
#9606=ORIENTED_EDGE('',*,*,#7059,.T.);
#9607=ORIENTED_EDGE('',*,*,#7060,.F.);
#9608=ORIENTED_EDGE('',*,*,#7061,.F.);
#9609=ORIENTED_EDGE('',*,*,#7045,.F.);
#9610=ORIENTED_EDGE('',*,*,#7061,.T.);
#9611=ORIENTED_EDGE('',*,*,#7062,.F.);
#9612=ORIENTED_EDGE('',*,*,#7063,.F.);
#9613=ORIENTED_EDGE('',*,*,#7046,.F.);
#9614=ORIENTED_EDGE('',*,*,#6863,.T.);
#9615=ORIENTED_EDGE('',*,*,#7048,.T.);
#9616=ORIENTED_EDGE('',*,*,#7035,.F.);
#9617=ORIENTED_EDGE('',*,*,#7063,.T.);
#9618=ORIENTED_EDGE('',*,*,#7064,.F.);
#9619=ORIENTED_EDGE('',*,*,#7033,.T.);
#9620=ORIENTED_EDGE('',*,*,#6952,.T.);
#9621=ORIENTED_EDGE('',*,*,#6914,.T.);
#9622=ORIENTED_EDGE('',*,*,#7064,.T.);
#9623=ORIENTED_EDGE('',*,*,#7062,.T.);
#9624=ORIENTED_EDGE('',*,*,#7060,.T.);
#9625=ORIENTED_EDGE('',*,*,#7058,.T.);
#9626=ORIENTED_EDGE('',*,*,#7056,.T.);
#9627=ORIENTED_EDGE('',*,*,#7054,.T.);
#9628=ORIENTED_EDGE('',*,*,#7052,.T.);
#9629=ORIENTED_EDGE('',*,*,#7017,.T.);
#9630=ORIENTED_EDGE('',*,*,#7022,.T.);
#9631=ORIENTED_EDGE('',*,*,#7026,.T.);
#9632=ORIENTED_EDGE('',*,*,#7028,.T.);
#9633=ORIENTED_EDGE('',*,*,#7030,.T.);
#9634=ORIENTED_EDGE('',*,*,#7032,.T.);
#9635=ORIENTED_EDGE('',*,*,#7034,.T.);
#9636=ORIENTED_EDGE('',*,*,#6874,.T.);
#9637=ORIENTED_EDGE('',*,*,#6909,.T.);
#9638=ORIENTED_EDGE('',*,*,#6943,.T.);
#9639=ORIENTED_EDGE('',*,*,#7065,.T.);
#9640=ORIENTED_EDGE('',*,*,#7066,.F.);
#9641=ORIENTED_EDGE('',*,*,#7067,.F.);
#9642=ORIENTED_EDGE('',*,*,#7068,.F.);
#9643=ORIENTED_EDGE('',*,*,#7069,.T.);
#9644=ORIENTED_EDGE('',*,*,#6942,.T.);
#9645=ORIENTED_EDGE('',*,*,#7070,.T.);
#9646=ORIENTED_EDGE('',*,*,#7071,.F.);
#9647=ORIENTED_EDGE('',*,*,#7065,.F.);
#9648=ORIENTED_EDGE('',*,*,#6875,.T.);
#9649=ORIENTED_EDGE('',*,*,#7069,.F.);
#9650=ORIENTED_EDGE('',*,*,#7072,.F.);
#9651=ORIENTED_EDGE('',*,*,#7073,.T.);
#9652=ORIENTED_EDGE('',*,*,#6941,.T.);
#9653=ORIENTED_EDGE('',*,*,#7074,.T.);
#9654=ORIENTED_EDGE('',*,*,#7075,.F.);
#9655=ORIENTED_EDGE('',*,*,#7070,.F.);
#9656=ORIENTED_EDGE('',*,*,#6940,.T.);
#9657=ORIENTED_EDGE('',*,*,#7076,.T.);
#9658=ORIENTED_EDGE('',*,*,#7077,.F.);
#9659=ORIENTED_EDGE('',*,*,#7074,.F.);
#9660=ORIENTED_EDGE('',*,*,#6939,.T.);
#9661=ORIENTED_EDGE('',*,*,#7078,.T.);
#9662=ORIENTED_EDGE('',*,*,#7079,.F.);
#9663=ORIENTED_EDGE('',*,*,#7076,.F.);
#9664=ORIENTED_EDGE('',*,*,#6938,.T.);
#9665=ORIENTED_EDGE('',*,*,#7080,.T.);
#9666=ORIENTED_EDGE('',*,*,#7081,.F.);
#9667=ORIENTED_EDGE('',*,*,#7078,.F.);
#9668=ORIENTED_EDGE('',*,*,#6937,.T.);
#9669=ORIENTED_EDGE('',*,*,#7082,.F.);
#9670=ORIENTED_EDGE('',*,*,#7083,.F.);
#9671=ORIENTED_EDGE('',*,*,#7080,.F.);
#9672=ORIENTED_EDGE('',*,*,#7084,.T.);
#9673=ORIENTED_EDGE('',*,*,#7085,.T.);
#9674=ORIENTED_EDGE('',*,*,#7086,.T.);
#9675=ORIENTED_EDGE('',*,*,#7087,.T.);
#9676=ORIENTED_EDGE('',*,*,#7088,.T.);
#9677=ORIENTED_EDGE('',*,*,#7089,.T.);
#9678=ORIENTED_EDGE('',*,*,#7072,.T.);
#9679=ORIENTED_EDGE('',*,*,#7068,.T.);
#9680=ORIENTED_EDGE('',*,*,#7090,.T.);
#9681=ORIENTED_EDGE('',*,*,#7091,.T.);
#9682=ORIENTED_EDGE('',*,*,#7092,.T.);
#9683=ORIENTED_EDGE('',*,*,#7093,.T.);
#9684=ORIENTED_EDGE('',*,*,#7094,.T.);
#9685=ORIENTED_EDGE('',*,*,#7095,.T.);
#9686=ORIENTED_EDGE('',*,*,#6880,.T.);
#9687=ORIENTED_EDGE('',*,*,#7096,.F.);
#9688=ORIENTED_EDGE('',*,*,#7085,.F.);
#9689=ORIENTED_EDGE('',*,*,#7097,.F.);
#9690=ORIENTED_EDGE('',*,*,#6879,.T.);
#9691=ORIENTED_EDGE('',*,*,#7098,.F.);
#9692=ORIENTED_EDGE('',*,*,#7086,.F.);
#9693=ORIENTED_EDGE('',*,*,#7096,.T.);
#9694=ORIENTED_EDGE('',*,*,#6878,.T.);
#9695=ORIENTED_EDGE('',*,*,#7099,.F.);
#9696=ORIENTED_EDGE('',*,*,#7087,.F.);
#9697=ORIENTED_EDGE('',*,*,#7098,.T.);
#9698=ORIENTED_EDGE('',*,*,#6877,.T.);
#9699=ORIENTED_EDGE('',*,*,#7100,.F.);
#9700=ORIENTED_EDGE('',*,*,#7088,.F.);
#9701=ORIENTED_EDGE('',*,*,#7099,.T.);
#9702=ORIENTED_EDGE('',*,*,#6876,.T.);
#9703=ORIENTED_EDGE('',*,*,#7073,.F.);
#9704=ORIENTED_EDGE('',*,*,#7089,.F.);
#9705=ORIENTED_EDGE('',*,*,#7100,.T.);
#9706=ORIENTED_EDGE('',*,*,#7067,.T.);
#9707=ORIENTED_EDGE('',*,*,#7101,.F.);
#9708=ORIENTED_EDGE('',*,*,#7102,.F.);
#9709=ORIENTED_EDGE('',*,*,#7090,.F.);
#9710=ORIENTED_EDGE('',*,*,#7102,.T.);
#9711=ORIENTED_EDGE('',*,*,#7103,.F.);
#9712=ORIENTED_EDGE('',*,*,#7104,.F.);
#9713=ORIENTED_EDGE('',*,*,#7091,.F.);
#9714=ORIENTED_EDGE('',*,*,#7104,.T.);
#9715=ORIENTED_EDGE('',*,*,#7105,.F.);
#9716=ORIENTED_EDGE('',*,*,#7106,.F.);
#9717=ORIENTED_EDGE('',*,*,#7092,.F.);
#9718=ORIENTED_EDGE('',*,*,#7106,.T.);
#9719=ORIENTED_EDGE('',*,*,#7107,.F.);
#9720=ORIENTED_EDGE('',*,*,#7108,.F.);
#9721=ORIENTED_EDGE('',*,*,#7093,.F.);
#9722=ORIENTED_EDGE('',*,*,#7108,.T.);
#9723=ORIENTED_EDGE('',*,*,#7109,.F.);
#9724=ORIENTED_EDGE('',*,*,#7110,.F.);
#9725=ORIENTED_EDGE('',*,*,#7094,.F.);
#9726=ORIENTED_EDGE('',*,*,#7110,.T.);
#9727=ORIENTED_EDGE('',*,*,#7111,.F.);
#9728=ORIENTED_EDGE('',*,*,#7112,.F.);
#9729=ORIENTED_EDGE('',*,*,#7095,.F.);
#9730=ORIENTED_EDGE('',*,*,#6881,.T.);
#9731=ORIENTED_EDGE('',*,*,#7097,.T.);
#9732=ORIENTED_EDGE('',*,*,#7084,.F.);
#9733=ORIENTED_EDGE('',*,*,#7112,.T.);
#9734=ORIENTED_EDGE('',*,*,#7113,.F.);
#9735=ORIENTED_EDGE('',*,*,#7082,.T.);
#9736=ORIENTED_EDGE('',*,*,#6936,.T.);
#9737=ORIENTED_EDGE('',*,*,#6911,.T.);
#9738=ORIENTED_EDGE('',*,*,#7113,.T.);
#9739=ORIENTED_EDGE('',*,*,#7111,.T.);
#9740=ORIENTED_EDGE('',*,*,#7109,.T.);
#9741=ORIENTED_EDGE('',*,*,#7107,.T.);
#9742=ORIENTED_EDGE('',*,*,#7105,.T.);
#9743=ORIENTED_EDGE('',*,*,#7103,.T.);
#9744=ORIENTED_EDGE('',*,*,#7101,.T.);
#9745=ORIENTED_EDGE('',*,*,#7066,.T.);
#9746=ORIENTED_EDGE('',*,*,#7071,.T.);
#9747=ORIENTED_EDGE('',*,*,#7075,.T.);
#9748=ORIENTED_EDGE('',*,*,#7077,.T.);
#9749=ORIENTED_EDGE('',*,*,#7079,.T.);
#9750=ORIENTED_EDGE('',*,*,#7081,.T.);
#9751=ORIENTED_EDGE('',*,*,#7083,.T.);
#9752=ORIENTED_EDGE('',*,*,#6883,.T.);
#9753=ORIENTED_EDGE('',*,*,#6910,.T.);
#9754=ORIENTED_EDGE('',*,*,#6935,.T.);
#9755=ORIENTED_EDGE('',*,*,#7114,.T.);
#9756=ORIENTED_EDGE('',*,*,#7115,.F.);
#9757=ORIENTED_EDGE('',*,*,#7116,.F.);
#9758=ORIENTED_EDGE('',*,*,#7117,.F.);
#9759=ORIENTED_EDGE('',*,*,#7118,.T.);
#9760=ORIENTED_EDGE('',*,*,#6934,.T.);
#9761=ORIENTED_EDGE('',*,*,#7119,.T.);
#9762=ORIENTED_EDGE('',*,*,#7120,.F.);
#9763=ORIENTED_EDGE('',*,*,#7114,.F.);
#9764=ORIENTED_EDGE('',*,*,#6884,.T.);
#9765=ORIENTED_EDGE('',*,*,#7118,.F.);
#9766=ORIENTED_EDGE('',*,*,#7121,.F.);
#9767=ORIENTED_EDGE('',*,*,#7122,.T.);
#9768=ORIENTED_EDGE('',*,*,#6933,.T.);
#9769=ORIENTED_EDGE('',*,*,#7123,.T.);
#9770=ORIENTED_EDGE('',*,*,#7124,.F.);
#9771=ORIENTED_EDGE('',*,*,#7119,.F.);
#9772=ORIENTED_EDGE('',*,*,#6932,.T.);
#9773=ORIENTED_EDGE('',*,*,#7125,.T.);
#9774=ORIENTED_EDGE('',*,*,#7126,.F.);
#9775=ORIENTED_EDGE('',*,*,#7123,.F.);
#9776=ORIENTED_EDGE('',*,*,#6931,.T.);
#9777=ORIENTED_EDGE('',*,*,#7127,.T.);
#9778=ORIENTED_EDGE('',*,*,#7128,.F.);
#9779=ORIENTED_EDGE('',*,*,#7125,.F.);
#9780=ORIENTED_EDGE('',*,*,#6930,.T.);
#9781=ORIENTED_EDGE('',*,*,#7129,.T.);
#9782=ORIENTED_EDGE('',*,*,#7130,.F.);
#9783=ORIENTED_EDGE('',*,*,#7127,.F.);
#9784=ORIENTED_EDGE('',*,*,#6929,.T.);
#9785=ORIENTED_EDGE('',*,*,#7131,.F.);
#9786=ORIENTED_EDGE('',*,*,#7132,.F.);
#9787=ORIENTED_EDGE('',*,*,#7129,.F.);
#9788=ORIENTED_EDGE('',*,*,#7133,.T.);
#9789=ORIENTED_EDGE('',*,*,#7134,.T.);
#9790=ORIENTED_EDGE('',*,*,#7135,.T.);
#9791=ORIENTED_EDGE('',*,*,#7136,.T.);
#9792=ORIENTED_EDGE('',*,*,#7137,.T.);
#9793=ORIENTED_EDGE('',*,*,#7138,.T.);
#9794=ORIENTED_EDGE('',*,*,#7121,.T.);
#9795=ORIENTED_EDGE('',*,*,#7117,.T.);
#9796=ORIENTED_EDGE('',*,*,#7139,.T.);
#9797=ORIENTED_EDGE('',*,*,#7140,.T.);
#9798=ORIENTED_EDGE('',*,*,#7141,.T.);
#9799=ORIENTED_EDGE('',*,*,#7142,.T.);
#9800=ORIENTED_EDGE('',*,*,#7143,.T.);
#9801=ORIENTED_EDGE('',*,*,#7144,.T.);
#9802=ORIENTED_EDGE('',*,*,#6889,.T.);
#9803=ORIENTED_EDGE('',*,*,#7145,.F.);
#9804=ORIENTED_EDGE('',*,*,#7134,.F.);
#9805=ORIENTED_EDGE('',*,*,#7146,.F.);
#9806=ORIENTED_EDGE('',*,*,#6888,.T.);
#9807=ORIENTED_EDGE('',*,*,#7147,.F.);
#9808=ORIENTED_EDGE('',*,*,#7135,.F.);
#9809=ORIENTED_EDGE('',*,*,#7145,.T.);
#9810=ORIENTED_EDGE('',*,*,#6887,.T.);
#9811=ORIENTED_EDGE('',*,*,#7148,.F.);
#9812=ORIENTED_EDGE('',*,*,#7136,.F.);
#9813=ORIENTED_EDGE('',*,*,#7147,.T.);
#9814=ORIENTED_EDGE('',*,*,#6886,.T.);
#9815=ORIENTED_EDGE('',*,*,#7149,.F.);
#9816=ORIENTED_EDGE('',*,*,#7137,.F.);
#9817=ORIENTED_EDGE('',*,*,#7148,.T.);
#9818=ORIENTED_EDGE('',*,*,#6885,.T.);
#9819=ORIENTED_EDGE('',*,*,#7122,.F.);
#9820=ORIENTED_EDGE('',*,*,#7138,.F.);
#9821=ORIENTED_EDGE('',*,*,#7149,.T.);
#9822=ORIENTED_EDGE('',*,*,#7116,.T.);
#9823=ORIENTED_EDGE('',*,*,#7150,.F.);
#9824=ORIENTED_EDGE('',*,*,#7151,.F.);
#9825=ORIENTED_EDGE('',*,*,#7139,.F.);
#9826=ORIENTED_EDGE('',*,*,#7151,.T.);
#9827=ORIENTED_EDGE('',*,*,#7152,.F.);
#9828=ORIENTED_EDGE('',*,*,#7153,.F.);
#9829=ORIENTED_EDGE('',*,*,#7140,.F.);
#9830=ORIENTED_EDGE('',*,*,#7153,.T.);
#9831=ORIENTED_EDGE('',*,*,#7154,.F.);
#9832=ORIENTED_EDGE('',*,*,#7155,.F.);
#9833=ORIENTED_EDGE('',*,*,#7141,.F.);
#9834=ORIENTED_EDGE('',*,*,#7155,.T.);
#9835=ORIENTED_EDGE('',*,*,#7156,.F.);
#9836=ORIENTED_EDGE('',*,*,#7157,.F.);
#9837=ORIENTED_EDGE('',*,*,#7142,.F.);
#9838=ORIENTED_EDGE('',*,*,#7157,.T.);
#9839=ORIENTED_EDGE('',*,*,#7158,.F.);
#9840=ORIENTED_EDGE('',*,*,#7159,.F.);
#9841=ORIENTED_EDGE('',*,*,#7143,.F.);
#9842=ORIENTED_EDGE('',*,*,#7159,.T.);
#9843=ORIENTED_EDGE('',*,*,#7160,.F.);
#9844=ORIENTED_EDGE('',*,*,#7161,.F.);
#9845=ORIENTED_EDGE('',*,*,#7144,.F.);
#9846=ORIENTED_EDGE('',*,*,#6890,.T.);
#9847=ORIENTED_EDGE('',*,*,#7146,.T.);
#9848=ORIENTED_EDGE('',*,*,#7133,.F.);
#9849=ORIENTED_EDGE('',*,*,#7161,.T.);
#9850=ORIENTED_EDGE('',*,*,#7162,.F.);
#9851=ORIENTED_EDGE('',*,*,#7131,.T.);
#9852=ORIENTED_EDGE('',*,*,#6928,.T.);
#9853=ORIENTED_EDGE('',*,*,#6901,.T.);
#9854=ORIENTED_EDGE('',*,*,#7162,.T.);
#9855=ORIENTED_EDGE('',*,*,#7160,.T.);
#9856=ORIENTED_EDGE('',*,*,#7158,.T.);
#9857=ORIENTED_EDGE('',*,*,#7156,.T.);
#9858=ORIENTED_EDGE('',*,*,#7154,.T.);
#9859=ORIENTED_EDGE('',*,*,#7152,.T.);
#9860=ORIENTED_EDGE('',*,*,#7150,.T.);
#9861=ORIENTED_EDGE('',*,*,#7115,.T.);
#9862=ORIENTED_EDGE('',*,*,#7120,.T.);
#9863=ORIENTED_EDGE('',*,*,#7124,.T.);
#9864=ORIENTED_EDGE('',*,*,#7126,.T.);
#9865=ORIENTED_EDGE('',*,*,#7128,.T.);
#9866=ORIENTED_EDGE('',*,*,#7130,.T.);
#9867=ORIENTED_EDGE('',*,*,#7132,.T.);
#9868=ORIENTED_EDGE('',*,*,#6865,.T.);
#9869=ORIENTED_EDGE('',*,*,#6913,.T.);
#9870=ORIENTED_EDGE('',*,*,#6951,.T.);
#9871=ORIENTED_EDGE('',*,*,#7163,.T.);
#9872=ORIENTED_EDGE('',*,*,#7164,.F.);
#9873=ORIENTED_EDGE('',*,*,#7165,.F.);
#9874=ORIENTED_EDGE('',*,*,#7166,.F.);
#9875=ORIENTED_EDGE('',*,*,#7167,.T.);
#9876=ORIENTED_EDGE('',*,*,#6950,.T.);
#9877=ORIENTED_EDGE('',*,*,#7168,.T.);
#9878=ORIENTED_EDGE('',*,*,#7169,.F.);
#9879=ORIENTED_EDGE('',*,*,#7163,.F.);
#9880=ORIENTED_EDGE('',*,*,#6866,.T.);
#9881=ORIENTED_EDGE('',*,*,#7167,.F.);
#9882=ORIENTED_EDGE('',*,*,#7170,.F.);
#9883=ORIENTED_EDGE('',*,*,#7171,.T.);
#9884=ORIENTED_EDGE('',*,*,#6949,.T.);
#9885=ORIENTED_EDGE('',*,*,#7172,.T.);
#9886=ORIENTED_EDGE('',*,*,#7173,.F.);
#9887=ORIENTED_EDGE('',*,*,#7168,.F.);
#9888=ORIENTED_EDGE('',*,*,#6948,.T.);
#9889=ORIENTED_EDGE('',*,*,#7174,.T.);
#9890=ORIENTED_EDGE('',*,*,#7175,.F.);
#9891=ORIENTED_EDGE('',*,*,#7172,.F.);
#9892=ORIENTED_EDGE('',*,*,#6947,.T.);
#9893=ORIENTED_EDGE('',*,*,#7176,.T.);
#9894=ORIENTED_EDGE('',*,*,#7177,.F.);
#9895=ORIENTED_EDGE('',*,*,#7174,.F.);
#9896=ORIENTED_EDGE('',*,*,#6946,.T.);
#9897=ORIENTED_EDGE('',*,*,#7178,.T.);
#9898=ORIENTED_EDGE('',*,*,#7179,.F.);
#9899=ORIENTED_EDGE('',*,*,#7176,.F.);
#9900=ORIENTED_EDGE('',*,*,#6945,.T.);
#9901=ORIENTED_EDGE('',*,*,#7180,.F.);
#9902=ORIENTED_EDGE('',*,*,#7181,.F.);
#9903=ORIENTED_EDGE('',*,*,#7178,.F.);
#9904=ORIENTED_EDGE('',*,*,#7182,.T.);
#9905=ORIENTED_EDGE('',*,*,#7183,.T.);
#9906=ORIENTED_EDGE('',*,*,#7184,.T.);
#9907=ORIENTED_EDGE('',*,*,#7185,.T.);
#9908=ORIENTED_EDGE('',*,*,#7186,.T.);
#9909=ORIENTED_EDGE('',*,*,#7187,.T.);
#9910=ORIENTED_EDGE('',*,*,#7170,.T.);
#9911=ORIENTED_EDGE('',*,*,#7166,.T.);
#9912=ORIENTED_EDGE('',*,*,#7188,.T.);
#9913=ORIENTED_EDGE('',*,*,#7189,.T.);
#9914=ORIENTED_EDGE('',*,*,#7190,.T.);
#9915=ORIENTED_EDGE('',*,*,#7191,.T.);
#9916=ORIENTED_EDGE('',*,*,#7192,.T.);
#9917=ORIENTED_EDGE('',*,*,#7193,.T.);
#9918=ORIENTED_EDGE('',*,*,#6871,.T.);
#9919=ORIENTED_EDGE('',*,*,#7194,.F.);
#9920=ORIENTED_EDGE('',*,*,#7183,.F.);
#9921=ORIENTED_EDGE('',*,*,#7195,.F.);
#9922=ORIENTED_EDGE('',*,*,#6870,.T.);
#9923=ORIENTED_EDGE('',*,*,#7196,.F.);
#9924=ORIENTED_EDGE('',*,*,#7184,.F.);
#9925=ORIENTED_EDGE('',*,*,#7194,.T.);
#9926=ORIENTED_EDGE('',*,*,#6869,.T.);
#9927=ORIENTED_EDGE('',*,*,#7197,.F.);
#9928=ORIENTED_EDGE('',*,*,#7185,.F.);
#9929=ORIENTED_EDGE('',*,*,#7196,.T.);
#9930=ORIENTED_EDGE('',*,*,#6868,.T.);
#9931=ORIENTED_EDGE('',*,*,#7198,.F.);
#9932=ORIENTED_EDGE('',*,*,#7186,.F.);
#9933=ORIENTED_EDGE('',*,*,#7197,.T.);
#9934=ORIENTED_EDGE('',*,*,#6867,.T.);
#9935=ORIENTED_EDGE('',*,*,#7171,.F.);
#9936=ORIENTED_EDGE('',*,*,#7187,.F.);
#9937=ORIENTED_EDGE('',*,*,#7198,.T.);
#9938=ORIENTED_EDGE('',*,*,#7165,.T.);
#9939=ORIENTED_EDGE('',*,*,#7199,.F.);
#9940=ORIENTED_EDGE('',*,*,#7200,.F.);
#9941=ORIENTED_EDGE('',*,*,#7188,.F.);
#9942=ORIENTED_EDGE('',*,*,#7200,.T.);
#9943=ORIENTED_EDGE('',*,*,#7201,.F.);
#9944=ORIENTED_EDGE('',*,*,#7202,.F.);
#9945=ORIENTED_EDGE('',*,*,#7189,.F.);
#9946=ORIENTED_EDGE('',*,*,#7202,.T.);
#9947=ORIENTED_EDGE('',*,*,#7203,.F.);
#9948=ORIENTED_EDGE('',*,*,#7204,.F.);
#9949=ORIENTED_EDGE('',*,*,#7190,.F.);
#9950=ORIENTED_EDGE('',*,*,#7204,.T.);
#9951=ORIENTED_EDGE('',*,*,#7205,.F.);
#9952=ORIENTED_EDGE('',*,*,#7206,.F.);
#9953=ORIENTED_EDGE('',*,*,#7191,.F.);
#9954=ORIENTED_EDGE('',*,*,#7206,.T.);
#9955=ORIENTED_EDGE('',*,*,#7207,.F.);
#9956=ORIENTED_EDGE('',*,*,#7208,.F.);
#9957=ORIENTED_EDGE('',*,*,#7192,.F.);
#9958=ORIENTED_EDGE('',*,*,#7208,.T.);
#9959=ORIENTED_EDGE('',*,*,#7209,.F.);
#9960=ORIENTED_EDGE('',*,*,#7210,.F.);
#9961=ORIENTED_EDGE('',*,*,#7193,.F.);
#9962=ORIENTED_EDGE('',*,*,#6872,.T.);
#9963=ORIENTED_EDGE('',*,*,#7195,.T.);
#9964=ORIENTED_EDGE('',*,*,#7182,.F.);
#9965=ORIENTED_EDGE('',*,*,#7210,.T.);
#9966=ORIENTED_EDGE('',*,*,#7211,.F.);
#9967=ORIENTED_EDGE('',*,*,#7180,.T.);
#9968=ORIENTED_EDGE('',*,*,#6944,.T.);
#9969=ORIENTED_EDGE('',*,*,#6907,.T.);
#9970=ORIENTED_EDGE('',*,*,#7211,.T.);
#9971=ORIENTED_EDGE('',*,*,#7209,.T.);
#9972=ORIENTED_EDGE('',*,*,#7207,.T.);
#9973=ORIENTED_EDGE('',*,*,#7205,.T.);
#9974=ORIENTED_EDGE('',*,*,#7203,.T.);
#9975=ORIENTED_EDGE('',*,*,#7201,.T.);
#9976=ORIENTED_EDGE('',*,*,#7199,.T.);
#9977=ORIENTED_EDGE('',*,*,#7164,.T.);
#9978=ORIENTED_EDGE('',*,*,#7169,.T.);
#9979=ORIENTED_EDGE('',*,*,#7173,.T.);
#9980=ORIENTED_EDGE('',*,*,#7175,.T.);
#9981=ORIENTED_EDGE('',*,*,#7177,.T.);
#9982=ORIENTED_EDGE('',*,*,#7179,.T.);
#9983=ORIENTED_EDGE('',*,*,#7181,.T.);
#9984=ORIENTED_EDGE('',*,*,#6847,.T.);
#9985=ORIENTED_EDGE('',*,*,#6916,.T.);
#9986=ORIENTED_EDGE('',*,*,#6919,.T.);
#9987=ORIENTED_EDGE('',*,*,#7212,.T.);
#9988=ORIENTED_EDGE('',*,*,#7213,.F.);
#9989=ORIENTED_EDGE('',*,*,#7214,.F.);
#9990=ORIENTED_EDGE('',*,*,#7215,.F.);
#9991=ORIENTED_EDGE('',*,*,#7216,.T.);
#9992=ORIENTED_EDGE('',*,*,#6966,.T.);
#9993=ORIENTED_EDGE('',*,*,#7217,.T.);
#9994=ORIENTED_EDGE('',*,*,#7218,.F.);
#9995=ORIENTED_EDGE('',*,*,#7212,.F.);
#9996=ORIENTED_EDGE('',*,*,#6848,.T.);
#9997=ORIENTED_EDGE('',*,*,#7216,.F.);
#9998=ORIENTED_EDGE('',*,*,#7219,.F.);
#9999=ORIENTED_EDGE('',*,*,#7220,.T.);
#10000=ORIENTED_EDGE('',*,*,#6965,.T.);
#10001=ORIENTED_EDGE('',*,*,#7221,.T.);
#10002=ORIENTED_EDGE('',*,*,#7222,.F.);
#10003=ORIENTED_EDGE('',*,*,#7217,.F.);
#10004=ORIENTED_EDGE('',*,*,#6964,.T.);
#10005=ORIENTED_EDGE('',*,*,#7223,.T.);
#10006=ORIENTED_EDGE('',*,*,#7224,.F.);
#10007=ORIENTED_EDGE('',*,*,#7221,.F.);
#10008=ORIENTED_EDGE('',*,*,#6963,.T.);
#10009=ORIENTED_EDGE('',*,*,#7225,.T.);
#10010=ORIENTED_EDGE('',*,*,#7226,.F.);
#10011=ORIENTED_EDGE('',*,*,#7223,.F.);
#10012=ORIENTED_EDGE('',*,*,#6962,.T.);
#10013=ORIENTED_EDGE('',*,*,#7227,.T.);
#10014=ORIENTED_EDGE('',*,*,#7228,.F.);
#10015=ORIENTED_EDGE('',*,*,#7225,.F.);
#10016=ORIENTED_EDGE('',*,*,#6961,.T.);
#10017=ORIENTED_EDGE('',*,*,#7229,.F.);
#10018=ORIENTED_EDGE('',*,*,#7230,.F.);
#10019=ORIENTED_EDGE('',*,*,#7227,.F.);
#10020=ORIENTED_EDGE('',*,*,#7231,.T.);
#10021=ORIENTED_EDGE('',*,*,#7232,.T.);
#10022=ORIENTED_EDGE('',*,*,#7233,.T.);
#10023=ORIENTED_EDGE('',*,*,#7234,.T.);
#10024=ORIENTED_EDGE('',*,*,#7235,.T.);
#10025=ORIENTED_EDGE('',*,*,#7236,.T.);
#10026=ORIENTED_EDGE('',*,*,#7219,.T.);
#10027=ORIENTED_EDGE('',*,*,#7215,.T.);
#10028=ORIENTED_EDGE('',*,*,#7237,.T.);
#10029=ORIENTED_EDGE('',*,*,#7238,.T.);
#10030=ORIENTED_EDGE('',*,*,#7239,.T.);
#10031=ORIENTED_EDGE('',*,*,#7240,.T.);
#10032=ORIENTED_EDGE('',*,*,#7241,.T.);
#10033=ORIENTED_EDGE('',*,*,#7242,.T.);
#10034=ORIENTED_EDGE('',*,*,#6853,.T.);
#10035=ORIENTED_EDGE('',*,*,#7243,.F.);
#10036=ORIENTED_EDGE('',*,*,#7232,.F.);
#10037=ORIENTED_EDGE('',*,*,#7244,.F.);
#10038=ORIENTED_EDGE('',*,*,#6852,.T.);
#10039=ORIENTED_EDGE('',*,*,#7245,.F.);
#10040=ORIENTED_EDGE('',*,*,#7233,.F.);
#10041=ORIENTED_EDGE('',*,*,#7243,.T.);
#10042=ORIENTED_EDGE('',*,*,#6851,.T.);
#10043=ORIENTED_EDGE('',*,*,#7246,.F.);
#10044=ORIENTED_EDGE('',*,*,#7234,.F.);
#10045=ORIENTED_EDGE('',*,*,#7245,.T.);
#10046=ORIENTED_EDGE('',*,*,#6850,.T.);
#10047=ORIENTED_EDGE('',*,*,#7247,.F.);
#10048=ORIENTED_EDGE('',*,*,#7235,.F.);
#10049=ORIENTED_EDGE('',*,*,#7246,.T.);
#10050=ORIENTED_EDGE('',*,*,#6849,.T.);
#10051=ORIENTED_EDGE('',*,*,#7220,.F.);
#10052=ORIENTED_EDGE('',*,*,#7236,.F.);
#10053=ORIENTED_EDGE('',*,*,#7247,.T.);
#10054=ORIENTED_EDGE('',*,*,#7214,.T.);
#10055=ORIENTED_EDGE('',*,*,#7248,.F.);
#10056=ORIENTED_EDGE('',*,*,#7249,.F.);
#10057=ORIENTED_EDGE('',*,*,#7237,.F.);
#10058=ORIENTED_EDGE('',*,*,#7249,.T.);
#10059=ORIENTED_EDGE('',*,*,#7250,.F.);
#10060=ORIENTED_EDGE('',*,*,#7251,.F.);
#10061=ORIENTED_EDGE('',*,*,#7238,.F.);
#10062=ORIENTED_EDGE('',*,*,#7251,.T.);
#10063=ORIENTED_EDGE('',*,*,#7252,.F.);
#10064=ORIENTED_EDGE('',*,*,#7253,.F.);
#10065=ORIENTED_EDGE('',*,*,#7239,.F.);
#10066=ORIENTED_EDGE('',*,*,#7253,.T.);
#10067=ORIENTED_EDGE('',*,*,#7254,.F.);
#10068=ORIENTED_EDGE('',*,*,#7255,.F.);
#10069=ORIENTED_EDGE('',*,*,#7240,.F.);
#10070=ORIENTED_EDGE('',*,*,#7255,.T.);
#10071=ORIENTED_EDGE('',*,*,#7256,.F.);
#10072=ORIENTED_EDGE('',*,*,#7257,.F.);
#10073=ORIENTED_EDGE('',*,*,#7241,.F.);
#10074=ORIENTED_EDGE('',*,*,#7257,.T.);
#10075=ORIENTED_EDGE('',*,*,#7258,.F.);
#10076=ORIENTED_EDGE('',*,*,#7259,.F.);
#10077=ORIENTED_EDGE('',*,*,#7242,.F.);
#10078=ORIENTED_EDGE('',*,*,#6854,.T.);
#10079=ORIENTED_EDGE('',*,*,#7244,.T.);
#10080=ORIENTED_EDGE('',*,*,#7231,.F.);
#10081=ORIENTED_EDGE('',*,*,#7259,.T.);
#10082=ORIENTED_EDGE('',*,*,#7260,.F.);
#10083=ORIENTED_EDGE('',*,*,#7229,.T.);
#10084=ORIENTED_EDGE('',*,*,#6960,.T.);
#10085=ORIENTED_EDGE('',*,*,#6904,.T.);
#10086=ORIENTED_EDGE('',*,*,#7260,.T.);
#10087=ORIENTED_EDGE('',*,*,#7258,.T.);
#10088=ORIENTED_EDGE('',*,*,#7256,.T.);
#10089=ORIENTED_EDGE('',*,*,#7254,.T.);
#10090=ORIENTED_EDGE('',*,*,#7252,.T.);
#10091=ORIENTED_EDGE('',*,*,#7250,.T.);
#10092=ORIENTED_EDGE('',*,*,#7248,.T.);
#10093=ORIENTED_EDGE('',*,*,#7213,.T.);
#10094=ORIENTED_EDGE('',*,*,#7218,.T.);
#10095=ORIENTED_EDGE('',*,*,#7222,.T.);
#10096=ORIENTED_EDGE('',*,*,#7224,.T.);
#10097=ORIENTED_EDGE('',*,*,#7226,.T.);
#10098=ORIENTED_EDGE('',*,*,#7228,.T.);
#10099=ORIENTED_EDGE('',*,*,#7230,.T.);
#10353=CYLINDRICAL_SURFACE('',#12108,0.817);
#10354=CYLINDRICAL_SURFACE('',#12110,0.817);
#10355=CYLINDRICAL_SURFACE('',#12112,0.817);
#10356=CYLINDRICAL_SURFACE('',#12114,0.817);
#10357=CYLINDRICAL_SURFACE('',#12116,0.817);
#10358=CYLINDRICAL_SURFACE('',#12118,0.817);
#10801=ADVANCED_FACE('',(#1459),#860,.F.);
#10802=ADVANCED_FACE('',(#1460),#10353,.T.);
#10803=ADVANCED_FACE('',(#1461),#10354,.T.);
#10804=ADVANCED_FACE('',(#1462),#10355,.T.);
#10805=ADVANCED_FACE('',(#1463),#10356,.T.);
#10806=ADVANCED_FACE('',(#1464),#10357,.T.);
#10807=ADVANCED_FACE('',(#1465),#10358,.T.);
#10808=ADVANCED_FACE('',(#1466),#861,.T.);
#10809=ADVANCED_FACE('',(#1467),#862,.T.);
#10810=ADVANCED_FACE('',(#1468),#863,.T.);
#10811=ADVANCED_FACE('',(#1469),#864,.T.);
#10812=ADVANCED_FACE('',(#1470),#865,.T.);
#10813=ADVANCED_FACE('',(#1471),#866,.T.);
#10814=ADVANCED_FACE('',(#1472),#867,.T.);
#10815=ADVANCED_FACE('',(#1473),#868,.T.);
#10816=ADVANCED_FACE('',(#1474),#869,.T.);
#10817=ADVANCED_FACE('',(#1475),#870,.T.);
#10818=ADVANCED_FACE('',(#1476),#871,.T.);
#10819=ADVANCED_FACE('',(#1477),#872,.T.);
#10820=ADVANCED_FACE('',(#1478),#873,.T.);
#10821=ADVANCED_FACE('',(#1479),#874,.T.);
#10822=ADVANCED_FACE('',(#1480),#875,.T.);
#10823=ADVANCED_FACE('',(#1481),#876,.T.);
#10824=ADVANCED_FACE('',(#1482),#877,.T.);
#10825=ADVANCED_FACE('',(#1483),#878,.T.);
#10826=ADVANCED_FACE('',(#1484),#879,.T.);
#10827=ADVANCED_FACE('',(#1485),#880,.T.);
#10828=ADVANCED_FACE('',(#1486),#881,.T.);
#10829=ADVANCED_FACE('',(#1487),#882,.T.);
#10830=ADVANCED_FACE('',(#1488),#883,.T.);
#10831=ADVANCED_FACE('',(#1489),#884,.T.);
#10832=ADVANCED_FACE('',(#1490),#885,.T.);
#10833=ADVANCED_FACE('',(#1491),#886,.T.);
#10834=ADVANCED_FACE('',(#1492),#887,.T.);
#10835=ADVANCED_FACE('',(#1493),#888,.T.);
#10836=ADVANCED_FACE('',(#1494),#889,.T.);
#10837=ADVANCED_FACE('',(#1495),#890,.T.);
#10838=ADVANCED_FACE('',(#1496),#891,.T.);
#10839=ADVANCED_FACE('',(#1497),#892,.T.);
#10840=ADVANCED_FACE('',(#1498),#893,.T.);
#10841=ADVANCED_FACE('',(#1499),#894,.T.);
#10842=ADVANCED_FACE('',(#1500),#895,.T.);
#10843=ADVANCED_FACE('',(#1501),#896,.T.);
#10844=ADVANCED_FACE('',(#1502),#897,.T.);
#10845=ADVANCED_FACE('',(#1503),#898,.T.);
#10846=ADVANCED_FACE('',(#1504),#899,.T.);
#10847=ADVANCED_FACE('',(#1505),#900,.T.);
#10848=ADVANCED_FACE('',(#1506),#901,.T.);
#10849=ADVANCED_FACE('',(#1507),#902,.T.);
#10850=ADVANCED_FACE('',(#1508),#903,.T.);
#10851=ADVANCED_FACE('',(#1509),#904,.T.);
#10852=ADVANCED_FACE('',(#1510),#905,.T.);
#10853=ADVANCED_FACE('',(#1511),#906,.T.);
#10854=ADVANCED_FACE('',(#1512),#907,.T.);
#10855=ADVANCED_FACE('',(#1513),#908,.T.);
#10856=ADVANCED_FACE('',(#1514),#909,.T.);
#10857=ADVANCED_FACE('',(#1515),#910,.T.);
#10858=ADVANCED_FACE('',(#1516),#911,.T.);
#10859=ADVANCED_FACE('',(#1517),#912,.T.);
#10860=ADVANCED_FACE('',(#1518),#913,.T.);
#10861=ADVANCED_FACE('',(#1519),#914,.T.);
#10862=ADVANCED_FACE('',(#1520),#915,.T.);
#10863=ADVANCED_FACE('',(#1521),#916,.T.);
#10864=ADVANCED_FACE('',(#1522),#917,.T.);
#10865=ADVANCED_FACE('',(#1523),#918,.T.);
#10866=ADVANCED_FACE('',(#1524),#919,.T.);
#10867=ADVANCED_FACE('',(#1525),#920,.T.);
#10868=ADVANCED_FACE('',(#1526),#921,.T.);
#10869=ADVANCED_FACE('',(#1527),#922,.T.);
#10870=ADVANCED_FACE('',(#1528),#923,.T.);
#10871=ADVANCED_FACE('',(#1529),#924,.T.);
#10872=ADVANCED_FACE('',(#1530),#925,.T.);
#10873=ADVANCED_FACE('',(#1531),#926,.T.);
#10874=ADVANCED_FACE('',(#1532),#927,.T.);
#10875=ADVANCED_FACE('',(#1533),#928,.T.);
#10876=ADVANCED_FACE('',(#1534),#929,.T.);
#10877=ADVANCED_FACE('',(#1535),#930,.T.);
#10878=ADVANCED_FACE('',(#1536),#931,.T.);
#10879=ADVANCED_FACE('',(#1537),#932,.T.);
#10880=ADVANCED_FACE('',(#1538),#933,.T.);
#10881=ADVANCED_FACE('',(#1539),#934,.T.);
#10882=ADVANCED_FACE('',(#1540),#935,.T.);
#10883=ADVANCED_FACE('',(#1541),#936,.T.);
#10884=ADVANCED_FACE('',(#1542),#937,.T.);
#10885=ADVANCED_FACE('',(#1543),#938,.T.);
#10886=ADVANCED_FACE('',(#1544),#939,.T.);
#10887=ADVANCED_FACE('',(#1545),#940,.T.);
#10888=ADVANCED_FACE('',(#1546),#941,.T.);
#10889=ADVANCED_FACE('',(#1547),#942,.T.);
#10890=ADVANCED_FACE('',(#1548),#943,.T.);
#10891=ADVANCED_FACE('',(#1549),#944,.T.);
#10892=ADVANCED_FACE('',(#1550),#945,.T.);
#10893=ADVANCED_FACE('',(#1551),#946,.T.);
#10894=ADVANCED_FACE('',(#1552),#947,.T.);
#10895=ADVANCED_FACE('',(#1553),#948,.T.);
#10896=ADVANCED_FACE('',(#1554),#949,.T.);
#10897=ADVANCED_FACE('',(#1555),#950,.T.);
#10898=ADVANCED_FACE('',(#1556),#951,.T.);
#10899=ADVANCED_FACE('',(#1557),#952,.T.);
#10900=ADVANCED_FACE('',(#1558),#953,.T.);
#10901=ADVANCED_FACE('',(#1559),#954,.T.);
#10902=ADVANCED_FACE('',(#1560),#955,.T.);
#10903=ADVANCED_FACE('',(#1561),#956,.T.);
#10904=ADVANCED_FACE('',(#1562),#957,.T.);
#10905=ADVANCED_FACE('',(#1563),#958,.T.);
#10906=ADVANCED_FACE('',(#1564),#959,.T.);
#10907=ADVANCED_FACE('',(#1565),#960,.T.);
#10908=ADVANCED_FACE('',(#1566),#961,.T.);
#10909=ADVANCED_FACE('',(#1567),#962,.T.);
#10910=ADVANCED_FACE('',(#1568),#963,.T.);
#10911=ADVANCED_FACE('',(#1569),#964,.T.);
#10912=ADVANCED_FACE('',(#1570),#965,.T.);
#10913=ADVANCED_FACE('',(#1571),#966,.T.);
#10914=ADVANCED_FACE('',(#1572),#967,.T.);
#10915=ADVANCED_FACE('',(#1573),#968,.T.);
#10916=ADVANCED_FACE('',(#1574),#969,.T.);
#10917=ADVANCED_FACE('',(#1575),#970,.T.);
#10918=ADVANCED_FACE('',(#1576),#971,.T.);
#10919=ADVANCED_FACE('',(#1577),#972,.T.);
#10920=ADVANCED_FACE('',(#1578),#973,.T.);
#10921=ADVANCED_FACE('',(#1579),#974,.T.);
#10922=ADVANCED_FACE('',(#1580),#975,.T.);
#10923=ADVANCED_FACE('',(#1581),#976,.T.);
#10924=ADVANCED_FACE('',(#1582),#977,.T.);
#10925=ADVANCED_FACE('',(#1583),#978,.T.);
#10926=ADVANCED_FACE('',(#1584),#979,.T.);
#10927=ADVANCED_FACE('',(#1585),#980,.T.);
#10928=ADVANCED_FACE('',(#1586),#981,.T.);
#10929=ADVANCED_FACE('',(#1587),#982,.T.);
#10930=ADVANCED_FACE('',(#1588),#983,.T.);
#10931=ADVANCED_FACE('',(#1589),#984,.T.);
#10932=ADVANCED_FACE('',(#1590),#985,.T.);
#10933=ADVANCED_FACE('',(#1591),#986,.T.);
#10934=ADVANCED_FACE('',(#1592),#987,.T.);
#10935=ADVANCED_FACE('',(#1593),#988,.T.);
#10936=ADVANCED_FACE('',(#1594),#989,.T.);
#10937=ADVANCED_FACE('',(#1595),#990,.T.);
#10938=ADVANCED_FACE('',(#1596),#991,.T.);
#10939=ADVANCED_FACE('',(#1597),#992,.T.);
#10940=ADVANCED_FACE('',(#1598),#993,.T.);
#11015=CLOSED_SHELL('',(#10801,#10802,#10803,#10804,#10805,#10806,#10807,
#10808,#10809,#10810,#10811,#10812,#10813,#10814,#10815,#10816,#10817,#10818,
#10819,#10820,#10821,#10822,#10823,#10824,#10825,#10826,#10827,#10828,#10829,
#10830,#10831,#10832,#10833,#10834,#10835,#10836,#10837,#10838,#10839,#10840,
#10841,#10842,#10843,#10844,#10845,#10846,#10847,#10848,#10849,#10850,#10851,
#10852,#10853,#10854,#10855,#10856,#10857,#10858,#10859,#10860,#10861,#10862,
#10863,#10864,#10865,#10866,#10867,#10868,#10869,#10870,#10871,#10872,#10873,
#10874,#10875,#10876,#10877,#10878,#10879,#10880,#10881,#10882,#10883,#10884,
#10885,#10886,#10887,#10888,#10889,#10890,#10891,#10892,#10893,#10894,#10895,
#10896,#10897,#10898,#10899,#10900,#10901,#10902,#10903,#10904,#10905,#10906,
#10907,#10908,#10909,#10910,#10911,#10912,#10913,#10914,#10915,#10916,#10917,
#10918,#10919,#10920,#10921,#10922,#10923,#10924,#10925,#10926,#10927,#10928,
#10929,#10930,#10931,#10932,#10933,#10934,#10935,#10936,#10937,#10938,#10939,
#10940));
#12100=AXIS2_PLACEMENT_3D('',#18251,#14480,#14481);
#12101=AXIS2_PLACEMENT_3D('',#18252,#14482,#14483);
#12102=AXIS2_PLACEMENT_3D('',#18271,#14492,#14493);
#12103=AXIS2_PLACEMENT_3D('',#18289,#14502,#14503);
#12104=AXIS2_PLACEMENT_3D('',#18307,#14512,#14513);
#12105=AXIS2_PLACEMENT_3D('',#18325,#14522,#14523);
#12106=AXIS2_PLACEMENT_3D('',#18343,#14532,#14533);
#12107=AXIS2_PLACEMENT_3D('',#18360,#14542,#14543);
#12108=AXIS2_PLACEMENT_3D('',#18361,#14544,#14545);
#12109=AXIS2_PLACEMENT_3D('',#18365,#14547,#14548);
#12110=AXIS2_PLACEMENT_3D('',#18367,#14550,#14551);
#12111=AXIS2_PLACEMENT_3D('',#18371,#14553,#14554);
#12112=AXIS2_PLACEMENT_3D('',#18373,#14556,#14557);
#12113=AXIS2_PLACEMENT_3D('',#18377,#14559,#14560);
#12114=AXIS2_PLACEMENT_3D('',#18379,#14562,#14563);
#12115=AXIS2_PLACEMENT_3D('',#18384,#14566,#14567);
#12116=AXIS2_PLACEMENT_3D('',#18385,#14568,#14569);
#12117=AXIS2_PLACEMENT_3D('',#18390,#14572,#14573);
#12118=AXIS2_PLACEMENT_3D('',#18391,#14574,#14575);
#12119=AXIS2_PLACEMENT_3D('',#18396,#14578,#14579);
#12120=AXIS2_PLACEMENT_3D('',#18397,#14580,#14581);
#12121=AXIS2_PLACEMENT_3D('',#18488,#14630,#14631);
#12122=AXIS2_PLACEMENT_3D('',#18498,#14637,#14638);
#12123=AXIS2_PLACEMENT_3D('',#18502,#14641,#14642);
#12124=AXIS2_PLACEMENT_3D('',#18506,#14645,#14646);
#12125=AXIS2_PLACEMENT_3D('',#18510,#14649,#14650);
#12126=AXIS2_PLACEMENT_3D('',#18514,#14653,#14654);
#12127=AXIS2_PLACEMENT_3D('',#18518,#14657,#14658);
#12128=AXIS2_PLACEMENT_3D('',#18522,#14661,#14662);
#12129=AXIS2_PLACEMENT_3D('',#18526,#14665,#14666);
#12130=AXIS2_PLACEMENT_3D('',#18550,#14679,#14680);
#12131=AXIS2_PLACEMENT_3D('',#18553,#14683,#14684);
#12132=AXIS2_PLACEMENT_3D('',#18555,#14686,#14687);
#12133=AXIS2_PLACEMENT_3D('',#18557,#14689,#14690);
#12134=AXIS2_PLACEMENT_3D('',#18559,#14692,#14693);
#12135=AXIS2_PLACEMENT_3D('',#18560,#14694,#14695);
#12136=AXIS2_PLACEMENT_3D('',#18564,#14698,#14699);
#12137=AXIS2_PLACEMENT_3D('',#18568,#14702,#14703);
#12138=AXIS2_PLACEMENT_3D('',#18572,#14706,#14707);
#12139=AXIS2_PLACEMENT_3D('',#18576,#14710,#14711);
#12140=AXIS2_PLACEMENT_3D('',#18580,#14714,#14715);
#12141=AXIS2_PLACEMENT_3D('',#18584,#14718,#14719);
#12142=AXIS2_PLACEMENT_3D('',#18586,#14721,#14722);
#12143=AXIS2_PLACEMENT_3D('',#18587,#14723,#14724);
#12144=AXIS2_PLACEMENT_3D('',#18597,#14730,#14731);
#12145=AXIS2_PLACEMENT_3D('',#18601,#14734,#14735);
#12146=AXIS2_PLACEMENT_3D('',#18605,#14738,#14739);
#12147=AXIS2_PLACEMENT_3D('',#18609,#14742,#14743);
#12148=AXIS2_PLACEMENT_3D('',#18613,#14746,#14747);
#12149=AXIS2_PLACEMENT_3D('',#18617,#14750,#14751);
#12150=AXIS2_PLACEMENT_3D('',#18621,#14754,#14755);
#12151=AXIS2_PLACEMENT_3D('',#18625,#14758,#14759);
#12152=AXIS2_PLACEMENT_3D('',#18649,#14772,#14773);
#12153=AXIS2_PLACEMENT_3D('',#18652,#14776,#14777);
#12154=AXIS2_PLACEMENT_3D('',#18654,#14779,#14780);
#12155=AXIS2_PLACEMENT_3D('',#18656,#14782,#14783);
#12156=AXIS2_PLACEMENT_3D('',#18658,#14785,#14786);
#12157=AXIS2_PLACEMENT_3D('',#18659,#14787,#14788);
#12158=AXIS2_PLACEMENT_3D('',#18663,#14791,#14792);
#12159=AXIS2_PLACEMENT_3D('',#18667,#14795,#14796);
#12160=AXIS2_PLACEMENT_3D('',#18671,#14799,#14800);
#12161=AXIS2_PLACEMENT_3D('',#18675,#14803,#14804);
#12162=AXIS2_PLACEMENT_3D('',#18679,#14807,#14808);
#12163=AXIS2_PLACEMENT_3D('',#18683,#14811,#14812);
#12164=AXIS2_PLACEMENT_3D('',#18685,#14814,#14815);
#12165=AXIS2_PLACEMENT_3D('',#18686,#14816,#14817);
#12166=AXIS2_PLACEMENT_3D('',#18696,#14823,#14824);
#12167=AXIS2_PLACEMENT_3D('',#18700,#14827,#14828);
#12168=AXIS2_PLACEMENT_3D('',#18704,#14831,#14832);
#12169=AXIS2_PLACEMENT_3D('',#18708,#14835,#14836);
#12170=AXIS2_PLACEMENT_3D('',#18712,#14839,#14840);
#12171=AXIS2_PLACEMENT_3D('',#18716,#14843,#14844);
#12172=AXIS2_PLACEMENT_3D('',#18720,#14847,#14848);
#12173=AXIS2_PLACEMENT_3D('',#18724,#14851,#14852);
#12174=AXIS2_PLACEMENT_3D('',#18748,#14865,#14866);
#12175=AXIS2_PLACEMENT_3D('',#18751,#14869,#14870);
#12176=AXIS2_PLACEMENT_3D('',#18753,#14872,#14873);
#12177=AXIS2_PLACEMENT_3D('',#18755,#14875,#14876);
#12178=AXIS2_PLACEMENT_3D('',#18757,#14878,#14879);
#12179=AXIS2_PLACEMENT_3D('',#18758,#14880,#14881);
#12180=AXIS2_PLACEMENT_3D('',#18762,#14884,#14885);
#12181=AXIS2_PLACEMENT_3D('',#18766,#14888,#14889);
#12182=AXIS2_PLACEMENT_3D('',#18770,#14892,#14893);
#12183=AXIS2_PLACEMENT_3D('',#18774,#14896,#14897);
#12184=AXIS2_PLACEMENT_3D('',#18778,#14900,#14901);
#12185=AXIS2_PLACEMENT_3D('',#18782,#14904,#14905);
#12186=AXIS2_PLACEMENT_3D('',#18784,#14907,#14908);
#12187=AXIS2_PLACEMENT_3D('',#18785,#14909,#14910);
#12188=AXIS2_PLACEMENT_3D('',#18795,#14916,#14917);
#12189=AXIS2_PLACEMENT_3D('',#18799,#14920,#14921);
#12190=AXIS2_PLACEMENT_3D('',#18803,#14924,#14925);
#12191=AXIS2_PLACEMENT_3D('',#18807,#14928,#14929);
#12192=AXIS2_PLACEMENT_3D('',#18811,#14932,#14933);
#12193=AXIS2_PLACEMENT_3D('',#18815,#14936,#14937);
#12194=AXIS2_PLACEMENT_3D('',#18819,#14940,#14941);
#12195=AXIS2_PLACEMENT_3D('',#18823,#14944,#14945);
#12196=AXIS2_PLACEMENT_3D('',#18847,#14958,#14959);
#12197=AXIS2_PLACEMENT_3D('',#18850,#14962,#14963);
#12198=AXIS2_PLACEMENT_3D('',#18852,#14965,#14966);
#12199=AXIS2_PLACEMENT_3D('',#18854,#14968,#14969);
#12200=AXIS2_PLACEMENT_3D('',#18856,#14971,#14972);
#12201=AXIS2_PLACEMENT_3D('',#18857,#14973,#14974);
#12202=AXIS2_PLACEMENT_3D('',#18861,#14977,#14978);
#12203=AXIS2_PLACEMENT_3D('',#18865,#14981,#14982);
#12204=AXIS2_PLACEMENT_3D('',#18869,#14985,#14986);
#12205=AXIS2_PLACEMENT_3D('',#18873,#14989,#14990);
#12206=AXIS2_PLACEMENT_3D('',#18877,#14993,#14994);
#12207=AXIS2_PLACEMENT_3D('',#18881,#14997,#14998);
#12208=AXIS2_PLACEMENT_3D('',#18883,#15000,#15001);
#12209=AXIS2_PLACEMENT_3D('',#18884,#15002,#15003);
#12210=AXIS2_PLACEMENT_3D('',#18894,#15009,#15010);
#12211=AXIS2_PLACEMENT_3D('',#18898,#15013,#15014);
#12212=AXIS2_PLACEMENT_3D('',#18902,#15017,#15018);
#12213=AXIS2_PLACEMENT_3D('',#18906,#15021,#15022);
#12214=AXIS2_PLACEMENT_3D('',#18910,#15025,#15026);
#12215=AXIS2_PLACEMENT_3D('',#18914,#15029,#15030);
#12216=AXIS2_PLACEMENT_3D('',#18918,#15033,#15034);
#12217=AXIS2_PLACEMENT_3D('',#18922,#15037,#15038);
#12218=AXIS2_PLACEMENT_3D('',#18946,#15051,#15052);
#12219=AXIS2_PLACEMENT_3D('',#18949,#15055,#15056);
#12220=AXIS2_PLACEMENT_3D('',#18951,#15058,#15059);
#12221=AXIS2_PLACEMENT_3D('',#18953,#15061,#15062);
#12222=AXIS2_PLACEMENT_3D('',#18955,#15064,#15065);
#12223=AXIS2_PLACEMENT_3D('',#18956,#15066,#15067);
#12224=AXIS2_PLACEMENT_3D('',#18960,#15070,#15071);
#12225=AXIS2_PLACEMENT_3D('',#18964,#15074,#15075);
#12226=AXIS2_PLACEMENT_3D('',#18968,#15078,#15079);
#12227=AXIS2_PLACEMENT_3D('',#18972,#15082,#15083);
#12228=AXIS2_PLACEMENT_3D('',#18976,#15086,#15087);
#12229=AXIS2_PLACEMENT_3D('',#18980,#15090,#15091);
#12230=AXIS2_PLACEMENT_3D('',#18982,#15093,#15094);
#12231=AXIS2_PLACEMENT_3D('',#18983,#15095,#15096);
#12232=AXIS2_PLACEMENT_3D('',#18993,#15102,#15103);
#12233=AXIS2_PLACEMENT_3D('',#18997,#15106,#15107);
#12234=AXIS2_PLACEMENT_3D('',#19001,#15110,#15111);
#12235=AXIS2_PLACEMENT_3D('',#19005,#15114,#15115);
#12236=AXIS2_PLACEMENT_3D('',#19009,#15118,#15119);
#12237=AXIS2_PLACEMENT_3D('',#19013,#15122,#15123);
#12238=AXIS2_PLACEMENT_3D('',#19017,#15126,#15127);
#12239=AXIS2_PLACEMENT_3D('',#19021,#15130,#15131);
#12240=AXIS2_PLACEMENT_3D('',#19045,#15144,#15145);
#12241=AXIS2_PLACEMENT_3D('',#19048,#15148,#15149);
#12242=AXIS2_PLACEMENT_3D('',#19050,#15151,#15152);
#12243=AXIS2_PLACEMENT_3D('',#19052,#15154,#15155);
#12244=AXIS2_PLACEMENT_3D('',#19054,#15157,#15158);
#12245=AXIS2_PLACEMENT_3D('',#19055,#15159,#15160);
#12246=AXIS2_PLACEMENT_3D('',#19059,#15163,#15164);
#12247=AXIS2_PLACEMENT_3D('',#19063,#15167,#15168);
#12248=AXIS2_PLACEMENT_3D('',#19067,#15171,#15172);
#12249=AXIS2_PLACEMENT_3D('',#19071,#15175,#15176);
#12250=AXIS2_PLACEMENT_3D('',#19075,#15179,#15180);
#12251=AXIS2_PLACEMENT_3D('',#19079,#15183,#15184);
#12252=AXIS2_PLACEMENT_3D('',#19081,#15186,#15187);
#14480=DIRECTION('axis',(0.,0.,1.));
#14481=DIRECTION('refdir',(1.,0.,0.));
#14482=DIRECTION('center_axis',(0.,1.,0.));
#14483=DIRECTION('ref_axis',(0.866025403784439,0.,-0.5));
#14484=DIRECTION('',(0.121869343405147,0.,0.992546151641322));
#14485=DIRECTION('',(0.994821748296033,0.,-0.101635078182804));
#14486=DIRECTION('',(0.998134798421867,0.,-0.0610485395348574));
#14487=DIRECTION('',(0.999792698085389,0.,-0.0203607675478923));
#14488=DIRECTION('',(0.999792698085388,0.,0.0203607675478936));
#14489=DIRECTION('',(0.998134798421867,0.,0.0610485395348586));
#14490=DIRECTION('',(0.994821748296033,0.,0.101635078182805));
#14491=DIRECTION('',(0.121869343405148,0.,-0.992546151641322));
#14492=DIRECTION('center_axis',(0.,-1.,0.));
#14493=DIRECTION('ref_axis',(0.866025403784439,0.,-0.5));
#14494=DIRECTION('',(-0.798635510047293,0.,0.601815023152048));
#14495=DIRECTION('',(0.585429433769943,0.,0.810723367170211));
#14496=DIRECTION('',(0.551936985312059,0.,0.833885822067168));
#14497=DIRECTION('',(0.517529290979719,0.,0.855665491286186));
#14498=DIRECTION('',(0.482263407105669,0.,0.876026258834079));
#14499=DIRECTION('',(0.446197813109808,0.,0.894934361602026));
#14500=DIRECTION('',(0.40939231452609,0.,0.912358445353015));
#14501=DIRECTION('',(0.92050485345244,0.,-0.390731128489274));
#14502=DIRECTION('center_axis',(0.,-1.,0.));
#14503=DIRECTION('ref_axis',(0.866025403784439,0.,-0.5));
#14504=DIRECTION('',(-0.92050485345244,0.,-0.390731128489274));
#14505=DIRECTION('',(-0.40939231452609,0.,0.912358445353015));
#14506=DIRECTION('',(-0.446197813109808,0.,0.894934361602025));
#14507=DIRECTION('',(-0.482263407105669,0.,0.876026258834078));
#14508=DIRECTION('',(-0.51752929097972,0.,0.855665491286185));
#14509=DIRECTION('',(-0.551936985312059,0.,0.833885822067168));
#14510=DIRECTION('',(-0.585429433769943,0.,0.810723367170211));
#14511=DIRECTION('',(0.798635510047293,0.,0.601815023152048));
#14512=DIRECTION('center_axis',(0.,-1.,0.));
#14513=DIRECTION('ref_axis',(0.866025403784439,0.,-0.5));
#14514=DIRECTION('',(-0.121869343405147,0.,-0.992546151641322));
#14515=DIRECTION('',(-0.994821748296033,0.,0.101635078182804));
#14516=DIRECTION('',(-0.998134798421867,0.,0.0610485395348577));
#14517=DIRECTION('',(-0.999792698085388,0.,0.0203607675478927));
#14518=DIRECTION('',(-0.999792698085389,0.,-0.0203607675478932));
#14519=DIRECTION('',(-0.998134798421867,0.,-0.0610485395348582));
#14520=DIRECTION('',(-0.994821748296033,0.,-0.101635078182805));
#14521=DIRECTION('',(-0.121869343405148,0.,0.992546151641322));
#14522=DIRECTION('center_axis',(0.,-1.,0.));
#14523=DIRECTION('ref_axis',(0.866025403784439,0.,-0.5));
#14524=DIRECTION('',(0.798635510047293,0.,-0.601815023152048));
#14525=DIRECTION('',(-0.585429433769943,0.,-0.810723367170211));
#14526=DIRECTION('',(-0.551936985312059,0.,-0.833885822067168));
#14527=DIRECTION('',(-0.517529290979719,0.,-0.855665491286186));
#14528=DIRECTION('',(-0.482263407105669,0.,-0.876026258834078));
#14529=DIRECTION('',(-0.446197813109808,0.,-0.894934361602026));
#14530=DIRECTION('',(-0.40939231452609,0.,-0.912358445353015));
#14531=DIRECTION('',(-0.92050485345244,0.,0.390731128489274));
#14532=DIRECTION('center_axis',(0.,-1.,0.));
#14533=DIRECTION('ref_axis',(0.866025403784439,0.,-0.5));
#14534=DIRECTION('',(0.92050485345244,0.,0.390731128489275));
#14535=DIRECTION('',(0.409392314526091,0.,-0.912358445353015));
#14536=DIRECTION('',(0.446197813109809,0.,-0.894934361602025));
#14537=DIRECTION('',(0.48226340710567,0.,-0.876026258834078));
#14538=DIRECTION('',(0.51752929097972,0.,-0.855665491286185));
#14539=DIRECTION('',(0.55193698531206,0.,-0.833885822067167));
#14540=DIRECTION('',(0.585429433769943,0.,-0.81072336717021));
#14541=DIRECTION('',(-0.798635510047292,0.,-0.601815023152049));
#14542=DIRECTION('center_axis',(0.,-1.,0.));
#14543=DIRECTION('ref_axis',(0.866025403784439,0.,-0.5));
#14544=DIRECTION('center_axis',(0.,1.,0.));
#14545=DIRECTION('ref_axis',(0.866025403784439,0.,-0.5));
#14546=DIRECTION('',(0.,-1.,0.));
#14547=DIRECTION('center_axis',(0.,1.,0.));
#14548=DIRECTION('ref_axis',(0.866025403784439,0.,-0.5));
#14549=DIRECTION('',(0.,1.,0.));
#14550=DIRECTION('center_axis',(0.,1.,0.));
#14551=DIRECTION('ref_axis',(0.866025403784439,0.,-0.5));
#14552=DIRECTION('',(0.,-1.,0.));
#14553=DIRECTION('center_axis',(0.,1.,0.));
#14554=DIRECTION('ref_axis',(0.866025403784439,0.,-0.5));
#14555=DIRECTION('',(0.,1.,0.));
#14556=DIRECTION('center_axis',(0.,1.,0.));
#14557=DIRECTION('ref_axis',(0.866025403784439,0.,-0.5));
#14558=DIRECTION('',(0.,-1.,0.));
#14559=DIRECTION('center_axis',(0.,1.,0.));
#14560=DIRECTION('ref_axis',(0.866025403784439,0.,-0.5));
#14561=DIRECTION('',(0.,1.,0.));
#14562=DIRECTION('center_axis',(0.,1.,0.));
#14563=DIRECTION('ref_axis',(0.866025403784439,0.,-0.5));
#14564=DIRECTION('',(0.,1.,0.));
#14565=DIRECTION('',(0.,-1.,0.));
#14566=DIRECTION('center_axis',(0.,1.,0.));
#14567=DIRECTION('ref_axis',(0.866025403784439,0.,-0.5));
#14568=DIRECTION('center_axis',(0.,1.,0.));
#14569=DIRECTION('ref_axis',(0.866025403784439,0.,-0.5));
#14570=DIRECTION('',(0.,1.,0.));
#14571=DIRECTION('',(0.,-1.,0.));
#14572=DIRECTION('center_axis',(0.,1.,0.));
#14573=DIRECTION('ref_axis',(0.866025403784439,0.,-0.5));
#14574=DIRECTION('center_axis',(0.,1.,0.));
#14575=DIRECTION('ref_axis',(0.866025403784439,0.,-0.5));
#14576=DIRECTION('',(0.,1.,0.));
#14577=DIRECTION('',(0.,-1.,0.));
#14578=DIRECTION('center_axis',(0.,1.,0.));
#14579=DIRECTION('ref_axis',(0.866025403784439,0.,-0.5));
#14580=DIRECTION('center_axis',(0.,1.,0.));
#14581=DIRECTION('ref_axis',(0.866025403784439,0.,-0.5));
#14582=DIRECTION('',(-0.121869343405147,0.,-0.992546151641322));
#14583=DIRECTION('',(0.798635510047292,0.,0.601815023152049));
#14584=DIRECTION('',(-0.585429433769943,0.,0.81072336717021));
#14585=DIRECTION('',(-0.55193698531206,0.,0.833885822067167));
#14586=DIRECTION('',(-0.51752929097972,0.,0.855665491286185));
#14587=DIRECTION('',(-0.48226340710567,0.,0.876026258834078));
#14588=DIRECTION('',(-0.446197813109809,0.,0.894934361602025));
#14589=DIRECTION('',(-0.409392314526091,0.,0.912358445353015));
#14590=DIRECTION('',(-0.92050485345244,0.,-0.390731128489275));
#14591=DIRECTION('',(0.92050485345244,0.,-0.390731128489274));
#14592=DIRECTION('',(0.40939231452609,0.,0.912358445353015));
#14593=DIRECTION('',(0.446197813109808,0.,0.894934361602026));
#14594=DIRECTION('',(0.482263407105669,0.,0.876026258834078));
#14595=DIRECTION('',(0.517529290979719,0.,0.855665491286186));
#14596=DIRECTION('',(0.551936985312059,0.,0.833885822067168));
#14597=DIRECTION('',(0.585429433769943,0.,0.810723367170211));
#14598=DIRECTION('',(-0.798635510047293,0.,0.601815023152048));
#14599=DIRECTION('',(0.121869343405148,0.,-0.992546151641322));
#14600=DIRECTION('',(0.994821748296033,0.,0.101635078182805));
#14601=DIRECTION('',(0.998134798421867,0.,0.0610485395348582));
#14602=DIRECTION('',(0.999792698085389,0.,0.0203607675478932));
#14603=DIRECTION('',(0.999792698085388,0.,-0.0203607675478927));
#14604=DIRECTION('',(0.998134798421867,0.,-0.0610485395348577));
#14605=DIRECTION('',(0.994821748296033,0.,-0.101635078182804));
#14606=DIRECTION('',(0.121869343405147,0.,0.992546151641322));
#14607=DIRECTION('',(-0.798635510047293,0.,-0.601815023152048));
#14608=DIRECTION('',(0.585429433769943,0.,-0.810723367170211));
#14609=DIRECTION('',(0.551936985312059,0.,-0.833885822067168));
#14610=DIRECTION('',(0.51752929097972,0.,-0.855665491286185));
#14611=DIRECTION('',(0.482263407105669,0.,-0.876026258834078));
#14612=DIRECTION('',(0.446197813109808,0.,-0.894934361602025));
#14613=DIRECTION('',(0.40939231452609,0.,-0.912358445353015));
#14614=DIRECTION('',(0.92050485345244,0.,0.390731128489274));
#14615=DIRECTION('',(-0.92050485345244,0.,0.390731128489274));
#14616=DIRECTION('',(-0.40939231452609,0.,-0.912358445353015));
#14617=DIRECTION('',(-0.446197813109808,0.,-0.894934361602026));
#14618=DIRECTION('',(-0.482263407105669,0.,-0.876026258834079));
#14619=DIRECTION('',(-0.517529290979719,0.,-0.855665491286186));
#14620=DIRECTION('',(-0.551936985312059,0.,-0.833885822067168));
#14621=DIRECTION('',(-0.585429433769943,0.,-0.810723367170211));
#14622=DIRECTION('',(0.798635510047293,0.,-0.601815023152048));
#14623=DIRECTION('',(-0.121869343405148,0.,0.992546151641322));
#14624=DIRECTION('',(-0.994821748296033,0.,-0.101635078182805));
#14625=DIRECTION('',(-0.998134798421867,0.,-0.0610485395348586));
#14626=DIRECTION('',(-0.999792698085388,0.,-0.0203607675478936));
#14627=DIRECTION('',(-0.999792698085389,0.,0.0203607675478923));
#14628=DIRECTION('',(-0.998134798421867,0.,0.0610485395348574));
#14629=DIRECTION('',(-0.994821748296033,0.,0.101635078182804));
#14630=DIRECTION('center_axis',(0.390731128489275,0.,-0.92050485345244));
#14631=DIRECTION('ref_axis',(-0.92050485345244,0.,-0.390731128489275));
#14632=DIRECTION('',(0.,1.,0.));
#14633=DIRECTION('',(-0.92050485345244,0.,-0.390731128489275));
#14634=DIRECTION('',(0.,1.,0.));
#14635=DIRECTION('',(0.92050485345244,0.,0.390731128489275));
#14636=DIRECTION('',(0.,1.,0.));
#14637=DIRECTION('center_axis',(-0.912358445353015,0.,-0.409392314526091));
#14638=DIRECTION('ref_axis',(-0.409392314526091,0.,0.912358445353015));
#14639=DIRECTION('',(0.,1.,0.));
#14640=DIRECTION('',(-0.409392314526091,0.,0.912358445353015));
#14641=DIRECTION('center_axis',(-0.912358445353015,0.,-0.409392314526091));
#14642=DIRECTION('ref_axis',(-0.409392314526091,0.,0.912358445353015));
#14643=DIRECTION('',(0.409392314526091,0.,-0.912358445353015));
#14644=DIRECTION('',(0.,1.,0.));
#14645=DIRECTION('center_axis',(-0.894934361602025,0.,-0.446197813109809));
#14646=DIRECTION('ref_axis',(-0.446197813109809,0.,0.894934361602025));
#14647=DIRECTION('',(0.,1.,0.));
#14648=DIRECTION('',(-0.446197813109809,0.,0.894934361602025));
#14649=DIRECTION('center_axis',(-0.876026258834078,0.,-0.48226340710567));
#14650=DIRECTION('ref_axis',(-0.48226340710567,0.,0.876026258834078));
#14651=DIRECTION('',(0.,1.,0.));
#14652=DIRECTION('',(-0.48226340710567,0.,0.876026258834078));
#14653=DIRECTION('center_axis',(-0.855665491286185,0.,-0.51752929097972));
#14654=DIRECTION('ref_axis',(-0.51752929097972,0.,0.855665491286185));
#14655=DIRECTION('',(0.,1.,0.));
#14656=DIRECTION('',(-0.51752929097972,0.,0.855665491286185));
#14657=DIRECTION('center_axis',(-0.833885822067167,0.,-0.55193698531206));
#14658=DIRECTION('ref_axis',(-0.55193698531206,0.,0.833885822067167));
#14659=DIRECTION('',(0.,1.,0.));
#14660=DIRECTION('',(-0.55193698531206,0.,0.833885822067167));
#14661=DIRECTION('center_axis',(-0.81072336717021,0.,-0.585429433769943));
#14662=DIRECTION('ref_axis',(-0.585429433769943,0.,0.81072336717021));
#14663=DIRECTION('',(0.,-1.,0.));
#14664=DIRECTION('',(-0.585429433769944,0.,0.81072336717021));
#14665=DIRECTION('center_axis',(0.,-1.,0.));
#14666=DIRECTION('ref_axis',(0.500000000000001,0.,-0.866025403784438));
#14667=DIRECTION('',(-0.798635510047292,0.,-0.601815023152049));
#14668=DIRECTION('',(0.585429433769944,0.,-0.81072336717021));
#14669=DIRECTION('',(0.55193698531206,0.,-0.833885822067167));
#14670=DIRECTION('',(0.51752929097972,0.,-0.855665491286185));
#14671=DIRECTION('',(0.48226340710567,0.,-0.876026258834078));
#14672=DIRECTION('',(0.446197813109809,0.,-0.894934361602025));
#14673=DIRECTION('',(-0.409392314526095,0.,0.912358445353013));
#14674=DIRECTION('',(-0.446197813109808,0.,0.894934361602026));
#14675=DIRECTION('',(-0.48226340710567,0.,0.876026258834078));
#14676=DIRECTION('',(-0.51752929097972,0.,0.855665491286185));
#14677=DIRECTION('',(-0.551936985312061,0.,0.833885822067167));
#14678=DIRECTION('',(-0.58542943376994,0.,0.810723367170213));
#14679=DIRECTION('center_axis',(-0.81072336717021,0.,-0.585429433769943));
#14680=DIRECTION('ref_axis',(-0.585429433769943,0.,0.81072336717021));
#14681=DIRECTION('',(0.,1.,0.));
#14682=DIRECTION('',(0.,-1.,0.));
#14683=DIRECTION('center_axis',(-0.833885822067167,0.,-0.55193698531206));
#14684=DIRECTION('ref_axis',(-0.55193698531206,0.,0.833885822067167));
#14685=DIRECTION('',(0.,1.,0.));
#14686=DIRECTION('center_axis',(-0.855665491286185,0.,-0.51752929097972));
#14687=DIRECTION('ref_axis',(-0.51752929097972,0.,0.855665491286185));
#14688=DIRECTION('',(0.,1.,0.));
#14689=DIRECTION('center_axis',(-0.876026258834078,0.,-0.48226340710567));
#14690=DIRECTION('ref_axis',(-0.48226340710567,0.,0.876026258834078));
#14691=DIRECTION('',(0.,1.,0.));
#14692=DIRECTION('center_axis',(-0.894934361602025,0.,-0.446197813109809));
#14693=DIRECTION('ref_axis',(-0.446197813109809,0.,0.894934361602025));
#14694=DIRECTION('center_axis',(0.912358445353013,0.,0.409392314526095));
#14695=DIRECTION('ref_axis',(0.409392314526095,0.,-0.912358445353013));
#14696=DIRECTION('',(0.409392314526095,0.,-0.912358445353013));
#14697=DIRECTION('',(0.,1.,0.));
#14698=DIRECTION('center_axis',(0.894934361602026,0.,0.446197813109808));
#14699=DIRECTION('ref_axis',(0.446197813109808,0.,-0.894934361602026));
#14700=DIRECTION('',(0.446197813109808,0.,-0.894934361602026));
#14701=DIRECTION('',(0.,1.,0.));
#14702=DIRECTION('center_axis',(0.876026258834078,0.,0.48226340710567));
#14703=DIRECTION('ref_axis',(0.48226340710567,0.,-0.876026258834078));
#14704=DIRECTION('',(0.48226340710567,0.,-0.876026258834078));
#14705=DIRECTION('',(0.,1.,0.));
#14706=DIRECTION('center_axis',(0.855665491286185,0.,0.51752929097972));
#14707=DIRECTION('ref_axis',(0.51752929097972,0.,-0.855665491286185));
#14708=DIRECTION('',(0.51752929097972,0.,-0.855665491286185));
#14709=DIRECTION('',(0.,1.,0.));
#14710=DIRECTION('center_axis',(0.833885822067167,0.,0.551936985312061));
#14711=DIRECTION('ref_axis',(0.551936985312061,0.,-0.833885822067167));
#14712=DIRECTION('',(0.551936985312061,0.,-0.833885822067167));
#14713=DIRECTION('',(0.,1.,0.));
#14714=DIRECTION('center_axis',(0.810723367170213,0.,0.58542943376994));
#14715=DIRECTION('ref_axis',(0.58542943376994,0.,-0.810723367170213));
#14716=DIRECTION('',(0.58542943376994,0.,-0.810723367170213));
#14717=DIRECTION('',(0.,1.,0.));
#14718=DIRECTION('center_axis',(-0.601815023152049,0.,0.798635510047292));
#14719=DIRECTION('ref_axis',(0.798635510047292,0.,0.601815023152049));
#14720=DIRECTION('',(0.798635510047292,0.,0.601815023152049));
#14721=DIRECTION('center_axis',(0.,1.,0.));
#14722=DIRECTION('ref_axis',(-0.500000000000001,0.,0.866025403784438));
#14723=DIRECTION('center_axis',(0.601815023152048,0.,0.798635510047293));
#14724=DIRECTION('ref_axis',(0.798635510047293,0.,-0.601815023152048));
#14725=DIRECTION('',(0.,1.,0.));
#14726=DIRECTION('',(0.798635510047293,0.,-0.601815023152048));
#14727=DIRECTION('',(0.,1.,0.));
#14728=DIRECTION('',(-0.798635510047293,0.,0.601815023152048));
#14729=DIRECTION('',(0.,1.,0.));
#14730=DIRECTION('center_axis',(0.810723367170211,0.,-0.585429433769943));
#14731=DIRECTION('ref_axis',(-0.585429433769943,0.,-0.810723367170211));
#14732=DIRECTION('',(0.,1.,0.));
#14733=DIRECTION('',(-0.585429433769943,0.,-0.810723367170211));
#14734=DIRECTION('center_axis',(0.810723367170211,0.,-0.585429433769943));
#14735=DIRECTION('ref_axis',(-0.585429433769943,0.,-0.810723367170211));
#14736=DIRECTION('',(0.585429433769943,0.,0.810723367170211));
#14737=DIRECTION('',(0.,1.,0.));
#14738=DIRECTION('center_axis',(0.833885822067168,0.,-0.551936985312059));
#14739=DIRECTION('ref_axis',(-0.551936985312059,0.,-0.833885822067168));
#14740=DIRECTION('',(0.,1.,0.));
#14741=DIRECTION('',(-0.551936985312059,0.,-0.833885822067168));
#14742=DIRECTION('center_axis',(0.855665491286186,0.,-0.517529290979719));
#14743=DIRECTION('ref_axis',(-0.517529290979719,0.,-0.855665491286186));
#14744=DIRECTION('',(0.,1.,0.));
#14745=DIRECTION('',(-0.517529290979719,0.,-0.855665491286186));
#14746=DIRECTION('center_axis',(0.876026258834078,0.,-0.482263407105669));
#14747=DIRECTION('ref_axis',(-0.482263407105669,0.,-0.876026258834079));
#14748=DIRECTION('',(0.,1.,0.));
#14749=DIRECTION('',(-0.482263407105669,0.,-0.876026258834079));
#14750=DIRECTION('center_axis',(0.894934361602026,0.,-0.446197813109808));
#14751=DIRECTION('ref_axis',(-0.446197813109808,0.,-0.894934361602026));
#14752=DIRECTION('',(0.,1.,0.));
#14753=DIRECTION('',(-0.446197813109808,0.,-0.894934361602026));
#14754=DIRECTION('center_axis',(0.912358445353015,0.,-0.40939231452609));
#14755=DIRECTION('ref_axis',(-0.40939231452609,0.,-0.912358445353015));
#14756=DIRECTION('',(0.,-1.,0.));
#14757=DIRECTION('',(-0.40939231452609,0.,-0.912358445353015));
#14758=DIRECTION('center_axis',(0.,-1.,0.));
#14759=DIRECTION('ref_axis',(0.5,0.,0.866025403784439));
#14760=DIRECTION('',(0.92050485345244,0.,-0.390731128489274));
#14761=DIRECTION('',(0.40939231452609,0.,0.912358445353015));
#14762=DIRECTION('',(0.446197813109808,0.,0.894934361602026));
#14763=DIRECTION('',(0.482263407105669,0.,0.876026258834079));
#14764=DIRECTION('',(0.517529290979719,0.,0.855665491286186));
#14765=DIRECTION('',(0.551936985312059,0.,0.833885822067168));
#14766=DIRECTION('',(-0.585429433769939,0.,-0.810723367170213));
#14767=DIRECTION('',(-0.55193698531206,0.,-0.833885822067167));
#14768=DIRECTION('',(-0.517529290979719,0.,-0.855665491286186));
#14769=DIRECTION('',(-0.482263407105669,0.,-0.876026258834078));
#14770=DIRECTION('',(-0.446197813109807,0.,-0.894934361602026));
#14771=DIRECTION('',(-0.409392314526094,0.,-0.912358445353014));
#14772=DIRECTION('center_axis',(0.912358445353015,0.,-0.40939231452609));
#14773=DIRECTION('ref_axis',(-0.40939231452609,0.,-0.912358445353015));
#14774=DIRECTION('',(0.,1.,0.));
#14775=DIRECTION('',(0.,-1.,0.));
#14776=DIRECTION('center_axis',(0.894934361602026,0.,-0.446197813109808));
#14777=DIRECTION('ref_axis',(-0.446197813109808,0.,-0.894934361602026));
#14778=DIRECTION('',(0.,1.,0.));
#14779=DIRECTION('center_axis',(0.876026258834078,0.,-0.482263407105669));
#14780=DIRECTION('ref_axis',(-0.482263407105669,0.,-0.876026258834079));
#14781=DIRECTION('',(0.,1.,0.));
#14782=DIRECTION('center_axis',(0.855665491286186,0.,-0.517529290979719));
#14783=DIRECTION('ref_axis',(-0.517529290979719,0.,-0.855665491286186));
#14784=DIRECTION('',(0.,1.,0.));
#14785=DIRECTION('center_axis',(0.833885822067168,0.,-0.551936985312059));
#14786=DIRECTION('ref_axis',(-0.551936985312059,0.,-0.833885822067168));
#14787=DIRECTION('center_axis',(-0.810723367170213,0.,0.585429433769939));
#14788=DIRECTION('ref_axis',(0.585429433769939,0.,0.810723367170213));
#14789=DIRECTION('',(0.585429433769939,0.,0.810723367170213));
#14790=DIRECTION('',(0.,1.,0.));
#14791=DIRECTION('center_axis',(-0.833885822067167,0.,0.55193698531206));
#14792=DIRECTION('ref_axis',(0.55193698531206,0.,0.833885822067167));
#14793=DIRECTION('',(0.55193698531206,0.,0.833885822067167));
#14794=DIRECTION('',(0.,1.,0.));
#14795=DIRECTION('center_axis',(-0.855665491286186,0.,0.517529290979719));
#14796=DIRECTION('ref_axis',(0.517529290979719,0.,0.855665491286186));
#14797=DIRECTION('',(0.517529290979719,0.,0.855665491286186));
#14798=DIRECTION('',(0.,1.,0.));
#14799=DIRECTION('center_axis',(-0.876026258834078,0.,0.482263407105669));
#14800=DIRECTION('ref_axis',(0.482263407105669,0.,0.876026258834078));
#14801=DIRECTION('',(0.482263407105669,0.,0.876026258834078));
#14802=DIRECTION('',(0.,1.,0.));
#14803=DIRECTION('center_axis',(-0.894934361602026,0.,0.446197813109807));
#14804=DIRECTION('ref_axis',(0.446197813109807,0.,0.894934361602026));
#14805=DIRECTION('',(0.446197813109807,0.,0.894934361602026));
#14806=DIRECTION('',(0.,1.,0.));
#14807=DIRECTION('center_axis',(-0.912358445353014,0.,0.409392314526094));
#14808=DIRECTION('ref_axis',(0.409392314526094,0.,0.912358445353014));
#14809=DIRECTION('',(0.409392314526094,0.,0.912358445353014));
#14810=DIRECTION('',(0.,1.,0.));
#14811=DIRECTION('center_axis',(-0.390731128489274,0.,-0.92050485345244));
#14812=DIRECTION('ref_axis',(-0.92050485345244,0.,0.390731128489274));
#14813=DIRECTION('',(-0.92050485345244,0.,0.390731128489274));
#14814=DIRECTION('center_axis',(0.,1.,0.));
#14815=DIRECTION('ref_axis',(-0.5,0.,-0.866025403784439));
#14816=DIRECTION('center_axis',(-0.992546151641322,0.,0.121869343405147));
#14817=DIRECTION('ref_axis',(0.121869343405147,0.,0.992546151641322));
#14818=DIRECTION('',(0.,1.,0.));
#14819=DIRECTION('',(0.121869343405147,0.,0.992546151641322));
#14820=DIRECTION('',(0.,1.,0.));
#14821=DIRECTION('',(-0.121869343405147,0.,-0.992546151641322));
#14822=DIRECTION('',(0.,1.,0.));
#14823=DIRECTION('center_axis',(0.101635078182804,0.,0.994821748296033));
#14824=DIRECTION('ref_axis',(0.994821748296033,0.,-0.101635078182804));
#14825=DIRECTION('',(0.,1.,0.));
#14826=DIRECTION('',(0.994821748296033,0.,-0.101635078182804));
#14827=DIRECTION('center_axis',(0.101635078182804,0.,0.994821748296033));
#14828=DIRECTION('ref_axis',(0.994821748296033,0.,-0.101635078182804));
#14829=DIRECTION('',(-0.994821748296033,0.,0.101635078182804));
#14830=DIRECTION('',(0.,1.,0.));
#14831=DIRECTION('center_axis',(0.0610485395348577,0.,0.998134798421867));
#14832=DIRECTION('ref_axis',(0.998134798421867,0.,-0.0610485395348577));
#14833=DIRECTION('',(0.,1.,0.));
#14834=DIRECTION('',(0.998134798421867,0.,-0.0610485395348577));
#14835=DIRECTION('center_axis',(0.0203607675478927,0.,0.999792698085389));
#14836=DIRECTION('ref_axis',(0.999792698085388,0.,-0.0203607675478927));
#14837=DIRECTION('',(0.,1.,0.));
#14838=DIRECTION('',(0.999792698085388,0.,-0.0203607675478927));
#14839=DIRECTION('center_axis',(-0.0203607675478932,0.,0.999792698085389));
#14840=DIRECTION('ref_axis',(0.999792698085389,0.,0.0203607675478932));
#14841=DIRECTION('',(0.,1.,0.));
#14842=DIRECTION('',(0.999792698085389,0.,0.0203607675478932));
#14843=DIRECTION('center_axis',(-0.0610485395348582,0.,0.998134798421867));
#14844=DIRECTION('ref_axis',(0.998134798421867,0.,0.0610485395348582));
#14845=DIRECTION('',(0.,1.,0.));
#14846=DIRECTION('',(0.998134798421867,0.,0.0610485395348582));
#14847=DIRECTION('center_axis',(-0.101635078182805,0.,0.994821748296033));
#14848=DIRECTION('ref_axis',(0.994821748296033,0.,0.101635078182805));
#14849=DIRECTION('',(0.,-1.,0.));
#14850=DIRECTION('',(0.994821748296033,0.,0.101635078182805));
#14851=DIRECTION('center_axis',(0.,-1.,0.));
#14852=DIRECTION('ref_axis',(-1.,0.,-2.22044604925031E-16));
#14853=DIRECTION('',(-0.121869343405148,0.,0.992546151641322));
#14854=DIRECTION('',(-0.994821748296033,0.,-0.101635078182805));
#14855=DIRECTION('',(-0.998134798421867,0.,-0.0610485395348582));
#14856=DIRECTION('',(-0.999792698085389,0.,-0.0203607675478932));
#14857=DIRECTION('',(-0.999792698085388,0.,0.0203607675478927));
#14858=DIRECTION('',(-0.998134798421867,0.,0.0610485395348577));
#14859=DIRECTION('',(0.994821748296033,0.,-0.1016350781828));
#14860=DIRECTION('',(0.998134798421867,0.,-0.0610485395348589));
#14861=DIRECTION('',(0.999792698085388,0.,-0.0203607675478925));
#14862=DIRECTION('',(0.999792698085389,0.,0.0203607675478929));
#14863=DIRECTION('',(0.998134798421867,0.,0.0610485395348593));
#14864=DIRECTION('',(0.994821748296033,0.,0.1016350781828));
#14865=DIRECTION('center_axis',(-0.101635078182805,0.,0.994821748296033));
#14866=DIRECTION('ref_axis',(0.994821748296033,0.,0.101635078182805));
#14867=DIRECTION('',(0.,1.,0.));
#14868=DIRECTION('',(0.,-1.,0.));
#14869=DIRECTION('center_axis',(-0.0610485395348582,0.,0.998134798421867));
#14870=DIRECTION('ref_axis',(0.998134798421867,0.,0.0610485395348582));
#14871=DIRECTION('',(0.,1.,0.));
#14872=DIRECTION('center_axis',(-0.0203607675478932,0.,0.999792698085389));
#14873=DIRECTION('ref_axis',(0.999792698085389,0.,0.0203607675478932));
#14874=DIRECTION('',(0.,1.,0.));
#14875=DIRECTION('center_axis',(0.0203607675478927,0.,0.999792698085389));
#14876=DIRECTION('ref_axis',(0.999792698085388,0.,-0.0203607675478927));
#14877=DIRECTION('',(0.,1.,0.));
#14878=DIRECTION('center_axis',(0.0610485395348577,0.,0.998134798421867));
#14879=DIRECTION('ref_axis',(0.998134798421867,0.,-0.0610485395348577));
#14880=DIRECTION('center_axis',(-0.1016350781828,0.,-0.994821748296033));
#14881=DIRECTION('ref_axis',(-0.994821748296033,0.,0.1016350781828));
#14882=DIRECTION('',(-0.994821748296033,0.,0.1016350781828));
#14883=DIRECTION('',(0.,1.,0.));
#14884=DIRECTION('center_axis',(-0.0610485395348589,0.,-0.998134798421867));
#14885=DIRECTION('ref_axis',(-0.998134798421867,0.,0.0610485395348589));
#14886=DIRECTION('',(-0.998134798421867,0.,0.0610485395348589));
#14887=DIRECTION('',(0.,1.,0.));
#14888=DIRECTION('center_axis',(-0.0203607675478925,0.,-0.999792698085389));
#14889=DIRECTION('ref_axis',(-0.999792698085388,0.,0.0203607675478925));
#14890=DIRECTION('',(-0.999792698085388,0.,0.0203607675478925));
#14891=DIRECTION('',(0.,1.,0.));
#14892=DIRECTION('center_axis',(0.0203607675478929,0.,-0.999792698085389));
#14893=DIRECTION('ref_axis',(-0.999792698085389,0.,-0.0203607675478929));
#14894=DIRECTION('',(-0.999792698085389,0.,-0.0203607675478929));
#14895=DIRECTION('',(0.,1.,0.));
#14896=DIRECTION('center_axis',(0.0610485395348593,0.,-0.998134798421867));
#14897=DIRECTION('ref_axis',(-0.998134798421867,0.,-0.0610485395348593));
#14898=DIRECTION('',(-0.998134798421867,0.,-0.0610485395348593));
#14899=DIRECTION('',(0.,1.,0.));
#14900=DIRECTION('center_axis',(0.1016350781828,0.,-0.994821748296033));
#14901=DIRECTION('ref_axis',(-0.994821748296033,0.,-0.1016350781828));
#14902=DIRECTION('',(-0.994821748296033,0.,-0.1016350781828));
#14903=DIRECTION('',(0.,1.,0.));
#14904=DIRECTION('center_axis',(0.992546151641322,0.,0.121869343405148));
#14905=DIRECTION('ref_axis',(0.121869343405148,0.,-0.992546151641322));
#14906=DIRECTION('',(0.121869343405148,0.,-0.992546151641322));
#14907=DIRECTION('center_axis',(0.,1.,0.));
#14908=DIRECTION('ref_axis',(1.,0.,2.22044604925031E-16));
#14909=DIRECTION('center_axis',(-0.601815023152048,0.,-0.798635510047293));
#14910=DIRECTION('ref_axis',(-0.798635510047293,0.,0.601815023152048));
#14911=DIRECTION('',(0.,1.,0.));
#14912=DIRECTION('',(-0.798635510047293,0.,0.601815023152048));
#14913=DIRECTION('',(0.,1.,0.));
#14914=DIRECTION('',(0.798635510047293,0.,-0.601815023152048));
#14915=DIRECTION('',(0.,1.,0.));
#14916=DIRECTION('center_axis',(-0.810723367170211,0.,0.585429433769943));
#14917=DIRECTION('ref_axis',(0.585429433769943,0.,0.810723367170211));
#14918=DIRECTION('',(0.,1.,0.));
#14919=DIRECTION('',(0.585429433769943,0.,0.810723367170211));
#14920=DIRECTION('center_axis',(-0.810723367170211,0.,0.585429433769943));
#14921=DIRECTION('ref_axis',(0.585429433769943,0.,0.810723367170211));
#14922=DIRECTION('',(-0.585429433769943,0.,-0.810723367170211));
#14923=DIRECTION('',(0.,1.,0.));
#14924=DIRECTION('center_axis',(-0.833885822067168,0.,0.551936985312059));
#14925=DIRECTION('ref_axis',(0.551936985312059,0.,0.833885822067168));
#14926=DIRECTION('',(0.,1.,0.));
#14927=DIRECTION('',(0.551936985312059,0.,0.833885822067168));
#14928=DIRECTION('center_axis',(-0.855665491286186,0.,0.517529290979719));
#14929=DIRECTION('ref_axis',(0.517529290979719,0.,0.855665491286186));
#14930=DIRECTION('',(0.,1.,0.));
#14931=DIRECTION('',(0.517529290979719,0.,0.855665491286186));
#14932=DIRECTION('center_axis',(-0.876026258834078,0.,0.482263407105669));
#14933=DIRECTION('ref_axis',(0.482263407105669,0.,0.876026258834078));
#14934=DIRECTION('',(0.,1.,0.));
#14935=DIRECTION('',(0.482263407105669,0.,0.876026258834078));
#14936=DIRECTION('center_axis',(-0.894934361602026,0.,0.446197813109808));
#14937=DIRECTION('ref_axis',(0.446197813109808,0.,0.894934361602026));
#14938=DIRECTION('',(0.,1.,0.));
#14939=DIRECTION('',(0.446197813109808,0.,0.894934361602026));
#14940=DIRECTION('center_axis',(-0.912358445353015,0.,0.40939231452609));
#14941=DIRECTION('ref_axis',(0.40939231452609,0.,0.912358445353015));
#14942=DIRECTION('',(0.,-1.,0.));
#14943=DIRECTION('',(0.40939231452609,0.,0.912358445353015));
#14944=DIRECTION('center_axis',(0.,-1.,0.));
#14945=DIRECTION('ref_axis',(-0.5,0.,-0.866025403784439));
#14946=DIRECTION('',(-0.92050485345244,0.,0.390731128489274));
#14947=DIRECTION('',(-0.40939231452609,0.,-0.912358445353015));
#14948=DIRECTION('',(-0.446197813109808,0.,-0.894934361602026));
#14949=DIRECTION('',(-0.482263407105669,0.,-0.876026258834078));
#14950=DIRECTION('',(-0.517529290979719,0.,-0.855665491286186));
#14951=DIRECTION('',(-0.551936985312059,0.,-0.833885822067168));
#14952=DIRECTION('',(0.585429433769939,0.,0.810723367170213));
#14953=DIRECTION('',(0.55193698531206,0.,0.833885822067167));
#14954=DIRECTION('',(0.517529290979719,0.,0.855665491286186));
#14955=DIRECTION('',(0.482263407105669,0.,0.876026258834078));
#14956=DIRECTION('',(0.446197813109807,0.,0.894934361602026));
#14957=DIRECTION('',(0.409392314526094,0.,0.912358445353014));
#14958=DIRECTION('center_axis',(-0.912358445353015,0.,0.40939231452609));
#14959=DIRECTION('ref_axis',(0.40939231452609,0.,0.912358445353015));
#14960=DIRECTION('',(0.,1.,0.));
#14961=DIRECTION('',(0.,-1.,0.));
#14962=DIRECTION('center_axis',(-0.894934361602026,0.,0.446197813109808));
#14963=DIRECTION('ref_axis',(0.446197813109808,0.,0.894934361602026));
#14964=DIRECTION('',(0.,1.,0.));
#14965=DIRECTION('center_axis',(-0.876026258834078,0.,0.482263407105669));
#14966=DIRECTION('ref_axis',(0.482263407105669,0.,0.876026258834078));
#14967=DIRECTION('',(0.,1.,0.));
#14968=DIRECTION('center_axis',(-0.855665491286186,0.,0.517529290979719));
#14969=DIRECTION('ref_axis',(0.517529290979719,0.,0.855665491286186));
#14970=DIRECTION('',(0.,1.,0.));
#14971=DIRECTION('center_axis',(-0.833885822067168,0.,0.551936985312059));
#14972=DIRECTION('ref_axis',(0.551936985312059,0.,0.833885822067168));
#14973=DIRECTION('center_axis',(0.810723367170213,0.,-0.585429433769939));
#14974=DIRECTION('ref_axis',(-0.585429433769939,0.,-0.810723367170213));
#14975=DIRECTION('',(-0.585429433769939,0.,-0.810723367170213));
#14976=DIRECTION('',(0.,1.,0.));
#14977=DIRECTION('center_axis',(0.833885822067167,0.,-0.55193698531206));
#14978=DIRECTION('ref_axis',(-0.55193698531206,0.,-0.833885822067167));
#14979=DIRECTION('',(-0.55193698531206,0.,-0.833885822067167));
#14980=DIRECTION('',(0.,1.,0.));
#14981=DIRECTION('center_axis',(0.855665491286186,0.,-0.517529290979719));
#14982=DIRECTION('ref_axis',(-0.517529290979719,0.,-0.855665491286186));
#14983=DIRECTION('',(-0.517529290979719,0.,-0.855665491286186));
#14984=DIRECTION('',(0.,1.,0.));
#14985=DIRECTION('center_axis',(0.876026258834078,0.,-0.482263407105669));
#14986=DIRECTION('ref_axis',(-0.482263407105669,0.,-0.876026258834078));
#14987=DIRECTION('',(-0.482263407105669,0.,-0.876026258834078));
#14988=DIRECTION('',(0.,1.,0.));
#14989=DIRECTION('center_axis',(0.894934361602026,0.,-0.446197813109807));
#14990=DIRECTION('ref_axis',(-0.446197813109807,0.,-0.894934361602026));
#14991=DIRECTION('',(-0.446197813109807,0.,-0.894934361602026));
#14992=DIRECTION('',(0.,1.,0.));
#14993=DIRECTION('center_axis',(0.912358445353014,0.,-0.409392314526094));
#14994=DIRECTION('ref_axis',(-0.409392314526094,0.,-0.912358445353014));
#14995=DIRECTION('',(-0.409392314526094,0.,-0.912358445353014));
#14996=DIRECTION('',(0.,1.,0.));
#14997=DIRECTION('center_axis',(0.390731128489274,0.,0.92050485345244));
#14998=DIRECTION('ref_axis',(0.92050485345244,0.,-0.390731128489274));
#14999=DIRECTION('',(0.92050485345244,0.,-0.390731128489274));
#15000=DIRECTION('center_axis',(0.,1.,0.));
#15001=DIRECTION('ref_axis',(0.5,0.,0.866025403784439));
#15002=DIRECTION('center_axis',(-0.390731128489274,0.,0.92050485345244));
#15003=DIRECTION('ref_axis',(0.92050485345244,0.,0.390731128489274));
#15004=DIRECTION('',(0.,1.,0.));
#15005=DIRECTION('',(0.92050485345244,0.,0.390731128489274));
#15006=DIRECTION('',(0.,1.,0.));
#15007=DIRECTION('',(-0.92050485345244,0.,-0.390731128489274));
#15008=DIRECTION('',(0.,1.,0.));
#15009=DIRECTION('center_axis',(0.912358445353015,0.,0.40939231452609));
#15010=DIRECTION('ref_axis',(0.40939231452609,0.,-0.912358445353015));
#15011=DIRECTION('',(0.,1.,0.));
#15012=DIRECTION('',(0.40939231452609,0.,-0.912358445353015));
#15013=DIRECTION('center_axis',(0.912358445353015,0.,0.40939231452609));
#15014=DIRECTION('ref_axis',(0.40939231452609,0.,-0.912358445353015));
#15015=DIRECTION('',(-0.40939231452609,0.,0.912358445353015));
#15016=DIRECTION('',(0.,1.,0.));
#15017=DIRECTION('center_axis',(0.894934361602025,0.,0.446197813109808));
#15018=DIRECTION('ref_axis',(0.446197813109808,0.,-0.894934361602025));
#15019=DIRECTION('',(0.,1.,0.));
#15020=DIRECTION('',(0.446197813109808,0.,-0.894934361602025));
#15021=DIRECTION('center_axis',(0.876026258834078,0.,0.482263407105669));
#15022=DIRECTION('ref_axis',(0.482263407105669,0.,-0.876026258834078));
#15023=DIRECTION('',(0.,1.,0.));
#15024=DIRECTION('',(0.482263407105669,0.,-0.876026258834078));
#15025=DIRECTION('center_axis',(0.855665491286185,0.,0.51752929097972));
#15026=DIRECTION('ref_axis',(0.51752929097972,0.,-0.855665491286185));
#15027=DIRECTION('',(0.,1.,0.));
#15028=DIRECTION('',(0.51752929097972,0.,-0.855665491286185));
#15029=DIRECTION('center_axis',(0.833885822067168,0.,0.551936985312059));
#15030=DIRECTION('ref_axis',(0.551936985312059,0.,-0.833885822067168));
#15031=DIRECTION('',(0.,1.,0.));
#15032=DIRECTION('',(0.551936985312059,0.,-0.833885822067167));
#15033=DIRECTION('center_axis',(0.810723367170211,0.,0.585429433769943));
#15034=DIRECTION('ref_axis',(0.585429433769943,0.,-0.810723367170211));
#15035=DIRECTION('',(0.,-1.,0.));
#15036=DIRECTION('',(0.585429433769943,0.,-0.810723367170211));
#15037=DIRECTION('center_axis',(0.,-1.,0.));
#15038=DIRECTION('ref_axis',(-0.5,0.,0.866025403784439));
#15039=DIRECTION('',(0.798635510047293,0.,0.601815023152048));
#15040=DIRECTION('',(-0.585429433769943,0.,0.810723367170211));
#15041=DIRECTION('',(-0.551936985312059,0.,0.833885822067167));
#15042=DIRECTION('',(-0.51752929097972,0.,0.855665491286185));
#15043=DIRECTION('',(-0.482263407105669,0.,0.876026258834078));
#15044=DIRECTION('',(-0.446197813109808,0.,0.894934361602025));
#15045=DIRECTION('',(0.409392314526094,0.,-0.912358445353013));
#15046=DIRECTION('',(0.446197813109807,0.,-0.894934361602026));
#15047=DIRECTION('',(0.48226340710567,0.,-0.876026258834078));
#15048=DIRECTION('',(0.517529290979719,0.,-0.855665491286185));
#15049=DIRECTION('',(0.55193698531206,0.,-0.833885822067167));
#15050=DIRECTION('',(0.58542943376994,0.,-0.810723367170213));
#15051=DIRECTION('center_axis',(0.810723367170211,0.,0.585429433769943));
#15052=DIRECTION('ref_axis',(0.585429433769943,0.,-0.810723367170211));
#15053=DIRECTION('',(0.,1.,0.));
#15054=DIRECTION('',(0.,-1.,0.));
#15055=DIRECTION('center_axis',(0.833885822067168,0.,0.551936985312059));
#15056=DIRECTION('ref_axis',(0.551936985312059,0.,-0.833885822067168));
#15057=DIRECTION('',(0.,1.,0.));
#15058=DIRECTION('center_axis',(0.855665491286185,0.,0.51752929097972));
#15059=DIRECTION('ref_axis',(0.51752929097972,0.,-0.855665491286185));
#15060=DIRECTION('',(0.,1.,0.));
#15061=DIRECTION('center_axis',(0.876026258834078,0.,0.482263407105669));
#15062=DIRECTION('ref_axis',(0.482263407105669,0.,-0.876026258834078));
#15063=DIRECTION('',(0.,1.,0.));
#15064=DIRECTION('center_axis',(0.894934361602025,0.,0.446197813109808));
#15065=DIRECTION('ref_axis',(0.446197813109808,0.,-0.894934361602025));
#15066=DIRECTION('center_axis',(-0.912358445353013,0.,-0.409392314526094));
#15067=DIRECTION('ref_axis',(-0.409392314526094,0.,0.912358445353013));
#15068=DIRECTION('',(-0.409392314526094,0.,0.912358445353013));
#15069=DIRECTION('',(0.,1.,0.));
#15070=DIRECTION('center_axis',(-0.894934361602026,0.,-0.446197813109807));
#15071=DIRECTION('ref_axis',(-0.446197813109807,0.,0.894934361602026));
#15072=DIRECTION('',(-0.446197813109807,0.,0.894934361602026));
#15073=DIRECTION('',(0.,1.,0.));
#15074=DIRECTION('center_axis',(-0.876026258834078,0.,-0.48226340710567));
#15075=DIRECTION('ref_axis',(-0.48226340710567,0.,0.876026258834078));
#15076=DIRECTION('',(-0.48226340710567,0.,0.876026258834078));
#15077=DIRECTION('',(0.,1.,0.));
#15078=DIRECTION('center_axis',(-0.855665491286185,0.,-0.517529290979719));
#15079=DIRECTION('ref_axis',(-0.517529290979719,0.,0.855665491286185));
#15080=DIRECTION('',(-0.517529290979719,0.,0.855665491286185));
#15081=DIRECTION('',(0.,1.,0.));
#15082=DIRECTION('center_axis',(-0.833885822067167,0.,-0.55193698531206));
#15083=DIRECTION('ref_axis',(-0.55193698531206,0.,0.833885822067167));
#15084=DIRECTION('',(-0.55193698531206,0.,0.833885822067167));
#15085=DIRECTION('',(0.,1.,0.));
#15086=DIRECTION('center_axis',(-0.810723367170213,0.,-0.585429433769939));
#15087=DIRECTION('ref_axis',(-0.585429433769939,0.,0.810723367170213));
#15088=DIRECTION('',(-0.58542943376994,0.,0.810723367170213));
#15089=DIRECTION('',(0.,1.,0.));
#15090=DIRECTION('center_axis',(0.601815023152048,0.,-0.798635510047293));
#15091=DIRECTION('ref_axis',(-0.798635510047293,0.,-0.601815023152048));
#15092=DIRECTION('',(-0.798635510047293,0.,-0.601815023152048));
#15093=DIRECTION('center_axis',(0.,1.,0.));
#15094=DIRECTION('ref_axis',(0.5,0.,-0.866025403784439));
#15095=DIRECTION('center_axis',(0.992546151641322,0.,-0.121869343405147));
#15096=DIRECTION('ref_axis',(-0.121869343405147,0.,-0.992546151641322));
#15097=DIRECTION('',(0.,1.,0.));
#15098=DIRECTION('',(-0.121869343405147,0.,-0.992546151641322));
#15099=DIRECTION('',(0.,1.,0.));
#15100=DIRECTION('',(0.121869343405147,0.,0.992546151641322));
#15101=DIRECTION('',(0.,1.,0.));
#15102=DIRECTION('center_axis',(-0.101635078182804,0.,-0.994821748296033));
#15103=DIRECTION('ref_axis',(-0.994821748296033,0.,0.101635078182804));
#15104=DIRECTION('',(0.,1.,0.));
#15105=DIRECTION('',(-0.994821748296033,0.,0.101635078182804));
#15106=DIRECTION('center_axis',(-0.101635078182804,0.,-0.994821748296033));
#15107=DIRECTION('ref_axis',(-0.994821748296033,0.,0.101635078182804));
#15108=DIRECTION('',(0.994821748296033,0.,-0.101635078182804));
#15109=DIRECTION('',(0.,1.,0.));
#15110=DIRECTION('center_axis',(-0.0610485395348574,0.,-0.998134798421867));
#15111=DIRECTION('ref_axis',(-0.998134798421867,0.,0.0610485395348574));
#15112=DIRECTION('',(0.,1.,0.));
#15113=DIRECTION('',(-0.998134798421867,0.,0.0610485395348574));
#15114=DIRECTION('center_axis',(-0.0203607675478923,0.,-0.999792698085389));
#15115=DIRECTION('ref_axis',(-0.999792698085389,0.,0.0203607675478923));
#15116=DIRECTION('',(0.,1.,0.));
#15117=DIRECTION('',(-0.999792698085389,0.,0.0203607675478923));
#15118=DIRECTION('center_axis',(0.0203607675478936,0.,-0.999792698085388));
#15119=DIRECTION('ref_axis',(-0.999792698085388,0.,-0.0203607675478936));
#15120=DIRECTION('',(0.,1.,0.));
#15121=DIRECTION('',(-0.999792698085388,0.,-0.0203607675478936));
#15122=DIRECTION('center_axis',(0.0610485395348586,0.,-0.998134798421867));
#15123=DIRECTION('ref_axis',(-0.998134798421867,0.,-0.0610485395348586));
#15124=DIRECTION('',(0.,1.,0.));
#15125=DIRECTION('',(-0.998134798421867,0.,-0.0610485395348586));
#15126=DIRECTION('center_axis',(0.101635078182805,0.,-0.994821748296033));
#15127=DIRECTION('ref_axis',(-0.994821748296033,0.,-0.101635078182805));
#15128=DIRECTION('',(0.,-1.,0.));
#15129=DIRECTION('',(-0.994821748296033,0.,-0.101635078182805));
#15130=DIRECTION('center_axis',(0.,-1.,0.));
#15131=DIRECTION('ref_axis',(1.,0.,6.10622663543836E-16));
#15132=DIRECTION('',(0.121869343405148,0.,-0.992546151641322));
#15133=DIRECTION('',(0.994821748296033,0.,0.101635078182805));
#15134=DIRECTION('',(0.998134798421867,0.,0.0610485395348586));
#15135=DIRECTION('',(0.999792698085388,0.,0.0203607675478936));
#15136=DIRECTION('',(0.999792698085389,0.,-0.0203607675478923));
#15137=DIRECTION('',(0.998134798421867,0.,-0.0610485395348574));
#15138=DIRECTION('',(-0.994821748296033,0.,0.1016350781828));
#15139=DIRECTION('',(-0.998134798421867,0.,0.0610485395348585));
#15140=DIRECTION('',(-0.999792698085389,0.,0.0203607675478921));
#15141=DIRECTION('',(-0.999792698085388,0.,-0.0203607675478933));
#15142=DIRECTION('',(-0.998134798421867,0.,-0.0610485395348597));
#15143=DIRECTION('',(-0.994821748296033,0.,-0.101635078182801));
#15144=DIRECTION('center_axis',(0.101635078182805,0.,-0.994821748296033));
#15145=DIRECTION('ref_axis',(-0.994821748296033,0.,-0.101635078182805));
#15146=DIRECTION('',(0.,1.,0.));
#15147=DIRECTION('',(0.,-1.,0.));
#15148=DIRECTION('center_axis',(0.0610485395348586,0.,-0.998134798421867));
#15149=DIRECTION('ref_axis',(-0.998134798421867,0.,-0.0610485395348586));
#15150=DIRECTION('',(0.,1.,0.));
#15151=DIRECTION('center_axis',(0.0203607675478936,0.,-0.999792698085388));
#15152=DIRECTION('ref_axis',(-0.999792698085388,0.,-0.0203607675478936));
#15153=DIRECTION('',(0.,1.,0.));
#15154=DIRECTION('center_axis',(-0.0203607675478923,0.,-0.999792698085389));
#15155=DIRECTION('ref_axis',(-0.999792698085389,0.,0.0203607675478923));
#15156=DIRECTION('',(0.,1.,0.));
#15157=DIRECTION('center_axis',(-0.0610485395348574,0.,-0.998134798421867));
#15158=DIRECTION('ref_axis',(-0.998134798421867,0.,0.0610485395348574));
#15159=DIRECTION('center_axis',(0.1016350781828,0.,0.994821748296033));
#15160=DIRECTION('ref_axis',(0.994821748296033,0.,-0.1016350781828));
#15161=DIRECTION('',(0.994821748296033,0.,-0.1016350781828));
#15162=DIRECTION('',(0.,1.,0.));
#15163=DIRECTION('center_axis',(0.0610485395348585,0.,0.998134798421867));
#15164=DIRECTION('ref_axis',(0.998134798421867,0.,-0.0610485395348585));
#15165=DIRECTION('',(0.998134798421867,0.,-0.0610485395348585));
#15166=DIRECTION('',(0.,1.,0.));
#15167=DIRECTION('center_axis',(0.0203607675478921,0.,0.999792698085389));
#15168=DIRECTION('ref_axis',(0.999792698085389,0.,-0.0203607675478921));
#15169=DIRECTION('',(0.999792698085389,0.,-0.0203607675478921));
#15170=DIRECTION('',(0.,1.,0.));
#15171=DIRECTION('center_axis',(-0.0203607675478933,0.,0.999792698085389));
#15172=DIRECTION('ref_axis',(0.999792698085388,0.,0.0203607675478933));
#15173=DIRECTION('',(0.999792698085388,0.,0.0203607675478933));
#15174=DIRECTION('',(0.,1.,0.));
#15175=DIRECTION('center_axis',(-0.0610485395348597,0.,0.998134798421867));
#15176=DIRECTION('ref_axis',(0.998134798421867,0.,0.0610485395348597));
#15177=DIRECTION('',(0.998134798421867,0.,0.0610485395348597));
#15178=DIRECTION('',(0.,1.,0.));
#15179=DIRECTION('center_axis',(-0.101635078182801,0.,0.994821748296033));
#15180=DIRECTION('ref_axis',(0.994821748296033,0.,0.101635078182801));
#15181=DIRECTION('',(0.994821748296033,0.,0.101635078182801));
#15182=DIRECTION('',(0.,1.,0.));
#15183=DIRECTION('center_axis',(-0.992546151641322,0.,-0.121869343405148));
#15184=DIRECTION('ref_axis',(-0.121869343405148,0.,0.992546151641322));
#15185=DIRECTION('',(-0.121869343405148,0.,0.992546151641322));
#15186=DIRECTION('center_axis',(0.,1.,0.));
#15187=DIRECTION('ref_axis',(-1.,0.,-6.10622663543836E-16));
#18251=CARTESIAN_POINT('',(0.,0.,0.));
#18252=CARTESIAN_POINT('Origin',(0.,-0.4,0.));
#18253=CARTESIAN_POINT('',(0.0994453842185998,-0.4,0.809917659739319));
#18254=CARTESIAN_POINT('',(0.099567253562005,-0.4,0.81091020589096));
#18255=CARTESIAN_POINT('',(0.0818108902278751,-0.4,0.666296231596819));
#18256=CARTESIAN_POINT('',(0.0663886785289718,-0.4,0.813294868644317));
#18257=CARTESIAN_POINT('',(0.091181207796194,-0.4,0.810761961965568));
#18258=CARTESIAN_POINT('',(0.0332218842499737,-0.4,0.815323436684413));
#18259=CARTESIAN_POINT('',(0.0580969799592227,-0.4,0.813802010654341));
#18260=CARTESIAN_POINT('',(-4.9960036108132E-16,-0.4,0.816));
#18261=CARTESIAN_POINT('',(0.0249164131874799,-0.4,0.81549257751331));
#18262=CARTESIAN_POINT('',(-0.0332218842499747,-0.4,0.815323436684413));
#18263=CARTESIAN_POINT('',(-0.00830547106249374,-0.4,0.815830859171103));
#18264=CARTESIAN_POINT('',(-0.0663886785289729,-0.4,0.813294868644317));
#18265=CARTESIAN_POINT('',(-0.0415135828197248,-0.4,0.814816294674389));
#18266=CARTESIAN_POINT('',(-0.0994453842186008,-0.4,0.809917659739319));
#18267=CARTESIAN_POINT('',(-0.074652854951381,-0.4,0.812450566418067));
#18268=CARTESIAN_POINT('',(-0.099567253562006,-0.4,0.81091020589096));
#18269=CARTESIAN_POINT('',(-0.0497226921093004,-0.4,0.404958829869659));
#18270=CARTESIAN_POINT('',(-0.652485211708638,-0.4,0.491682873915223));
#18271=CARTESIAN_POINT('Origin',(0.,-0.4,0.));
#18272=CARTESIAN_POINT('',(-0.651686576198591,-0.4,0.491081058892071));
#18273=CARTESIAN_POINT('',(-0.536124017894748,-0.4,0.40399842504197));
#18274=CARTESIAN_POINT('',(-0.671139677749021,-0.4,0.464141716451927));
#18275=CARTESIAN_POINT('',(-0.656549851586198,-0.4,0.484346223282036));
#18276=CARTESIAN_POINT('',(-0.689479866344548,-0.4,0.43643271406427));
#18277=CARTESIAN_POINT('',(-0.675724724897902,-0.4,0.457214465855013));
#18278=CARTESIAN_POINT('',(-0.706676729488102,-0.4,0.408));
#18279=CARTESIAN_POINT('',(-0.693779082130436,-0.4,0.429324535548202));
#18280=CARTESIAN_POINT('',(-0.722701750594522,-0.4,0.378890722620142));
#18281=CARTESIAN_POINT('',(-0.710682984764707,-0.4,0.400722680655036));
#18282=CARTESIAN_POINT('',(-0.737528356277993,-0.4,0.34915315219239));
#18283=CARTESIAN_POINT('',(-0.72640840201539,-0.4,0.371456330013204));
#18284=CARTESIAN_POINT('',(-0.751131960417191,-0.4,0.318836600847247));
#18285=CARTESIAN_POINT('',(-0.740929257312793,-0.4,0.341574014356103));
#18286=CARTESIAN_POINT('',(-0.752052465270644,-0.4,0.319227331975736));
#18287=CARTESIAN_POINT('',(-0.375565980208596,-0.4,0.159418300423624));
#18288=CARTESIAN_POINT('',(-0.752052465270644,-0.4,-0.319227331975737));
#18289=CARTESIAN_POINT('Origin',(0.,-0.4,0.));
#18290=CARTESIAN_POINT('',(-0.751131960417191,-0.4,-0.318836600847248));
#18291=CARTESIAN_POINT('',(-0.617934908122623,-0.4,-0.26229780655485));
#18292=CARTESIAN_POINT('',(-0.737528356277993,-0.4,-0.34915315219239));
#18293=CARTESIAN_POINT('',(-0.747731059382392,-0.4,-0.326415738683532));
#18294=CARTESIAN_POINT('',(-0.722701750594522,-0.4,-0.378890722620143));
#18295=CARTESIAN_POINT('',(-0.733821704857125,-0.4,-0.356587544799328));
#18296=CARTESIAN_POINT('',(-0.706676729488102,-0.4,-0.408));
#18297=CARTESIAN_POINT('',(-0.718695495317917,-0.4,-0.386168041965107));
#18298=CARTESIAN_POINT('',(-0.689479866344548,-0.4,-0.43643271406427));
#18299=CARTESIAN_POINT('',(-0.702377513702213,-0.4,-0.415108178516068));
#18300=CARTESIAN_POINT('',(-0.67113967774902,-0.4,-0.464141716451927));
#18301=CARTESIAN_POINT('',(-0.684894819195665,-0.4,-0.443359964661185));
#18302=CARTESIAN_POINT('',(-0.651686576198591,-0.4,-0.491081058892072));
#18303=CARTESIAN_POINT('',(-0.666276402361412,-0.4,-0.470876552061964));
#18304=CARTESIAN_POINT('',(-0.652485211708638,-0.4,-0.491682873915224));
#18305=CARTESIAN_POINT('',(-0.325843288099295,-0.4,-0.245540529446036));
#18306=CARTESIAN_POINT('',(-0.0995672535620054,-0.4,-0.81091020589096));
#18307=CARTESIAN_POINT('Origin',(0.,-0.4,0.));
#18308=CARTESIAN_POINT('',(-0.0994453842186002,-0.4,-0.809917659739319));
#18309=CARTESIAN_POINT('',(-0.0818108902278754,-0.4,-0.666296231596819));
#18310=CARTESIAN_POINT('',(-0.0663886785289722,-0.4,-0.813294868644317));
#18311=CARTESIAN_POINT('',(-0.0911812077961943,-0.4,-0.810761961965568));
#18312=CARTESIAN_POINT('',(-0.033221884249974,-0.4,-0.815323436684413));
#18313=CARTESIAN_POINT('',(-0.0580969799592231,-0.4,-0.813802010654341));
#18314=CARTESIAN_POINT('',(2.22044604925031E-16,-0.4,-0.816));
#18315=CARTESIAN_POINT('',(-0.0249164131874803,-0.4,-0.81549257751331));
#18316=CARTESIAN_POINT('',(0.0332218842499744,-0.4,-0.815323436684413));
#18317=CARTESIAN_POINT('',(0.00830547106249352,-0.4,-0.815830859171103));
#18318=CARTESIAN_POINT('',(0.0663886785289726,-0.4,-0.813294868644317));
#18319=CARTESIAN_POINT('',(0.0415135828197244,-0.4,-0.814816294674389));
#18320=CARTESIAN_POINT('',(0.0994453842186005,-0.4,-0.809917659739319));
#18321=CARTESIAN_POINT('',(0.0746528549513807,-0.4,-0.812450566418067));
#18322=CARTESIAN_POINT('',(0.0995672535620056,-0.4,-0.81091020589096));
#18323=CARTESIAN_POINT('',(0.0497226921093002,-0.4,-0.404958829869659));
#18324=CARTESIAN_POINT('',(0.652485211708638,-0.4,-0.491682873915223));
#18325=CARTESIAN_POINT('Origin',(0.,-0.4,0.));
#18326=CARTESIAN_POINT('',(0.651686576198591,-0.4,-0.491081058892071));
#18327=CARTESIAN_POINT('',(0.536124017894748,-0.4,-0.40399842504197));
#18328=CARTESIAN_POINT('',(0.67113967774902,-0.4,-0.464141716451927));
#18329=CARTESIAN_POINT('',(0.656549851586198,-0.4,-0.484346223282036));
#18330=CARTESIAN_POINT('',(0.689479866344548,-0.4,-0.43643271406427));
#18331=CARTESIAN_POINT('',(0.675724724897902,-0.4,-0.457214465855013));
#18332=CARTESIAN_POINT('',(0.706676729488102,-0.4,-0.408));
#18333=CARTESIAN_POINT('',(0.693779082130436,-0.4,-0.429324535548202));
#18334=CARTESIAN_POINT('',(0.722701750594522,-0.4,-0.378890722620142));
#18335=CARTESIAN_POINT('',(0.710682984764707,-0.4,-0.400722680655036));
#18336=CARTESIAN_POINT('',(0.737528356277993,-0.4,-0.34915315219239));
#18337=CARTESIAN_POINT('',(0.72640840201539,-0.4,-0.371456330013204));
#18338=CARTESIAN_POINT('',(0.751131960417191,-0.4,-0.318836600847247));
#18339=CARTESIAN_POINT('',(0.740929257312793,-0.4,-0.341574014356103));
#18340=CARTESIAN_POINT('',(0.752052465270644,-0.4,-0.319227331975737));
#18341=CARTESIAN_POINT('',(0.375565980208596,-0.4,-0.159418300423624));
#18342=CARTESIAN_POINT('',(0.752052465270643,-0.4,0.319227331975737));
#18343=CARTESIAN_POINT('Origin',(0.,-0.4,0.));
#18344=CARTESIAN_POINT('',(0.751131960417191,-0.4,0.318836600847248));
#18345=CARTESIAN_POINT('',(0.617934908122623,-0.4,0.26229780655485));
#18346=CARTESIAN_POINT('',(0.737528356277993,-0.4,0.349153152192391));
#18347=CARTESIAN_POINT('',(0.747731059382392,-0.4,0.326415738683533));
#18348=CARTESIAN_POINT('',(0.722701750594521,-0.4,0.378890722620143));
#18349=CARTESIAN_POINT('',(0.733821704857125,-0.4,0.356587544799328));
#18350=CARTESIAN_POINT('',(0.706676729488102,-0.4,0.408000000000001));
#18351=CARTESIAN_POINT('',(0.718695495317916,-0.4,0.386168041965108));
#18352=CARTESIAN_POINT('',(0.689479866344547,-0.4,0.436432714064271));
#18353=CARTESIAN_POINT('',(0.702377513702213,-0.4,0.415108178516068));
#18354=CARTESIAN_POINT('',(0.67113967774902,-0.4,0.464141716451928));
#18355=CARTESIAN_POINT('',(0.684894819195665,-0.4,0.443359964661185));
#18356=CARTESIAN_POINT('',(0.65168657619859,-0.4,0.491081058892072));
#18357=CARTESIAN_POINT('',(0.666276402361412,-0.4,0.470876552061965));
#18358=CARTESIAN_POINT('',(0.652485211708638,-0.4,0.491682873915224));
#18359=CARTESIAN_POINT('',(0.325843288099295,-0.4,0.245540529446036));
#18360=CARTESIAN_POINT('Origin',(0.,-0.4,0.));
#18361=CARTESIAN_POINT('Origin',(0.,0.,0.));
#18362=CARTESIAN_POINT('',(0.752052465270644,0.4,-0.319227331975737));
#18363=CARTESIAN_POINT('',(0.752052465270644,0.,-0.319227331975737));
#18364=CARTESIAN_POINT('',(0.752052465270643,0.4,0.319227331975737));
#18365=CARTESIAN_POINT('Origin',(0.,0.4,0.));
#18366=CARTESIAN_POINT('',(0.752052465270643,0.,0.319227331975737));
#18367=CARTESIAN_POINT('Origin',(0.,0.,0.));
#18368=CARTESIAN_POINT('',(-0.099567253562006,0.4,0.81091020589096));
#18369=CARTESIAN_POINT('',(-0.099567253562006,0.,0.81091020589096));
#18370=CARTESIAN_POINT('',(-0.652485211708638,0.4,0.491682873915223));
#18371=CARTESIAN_POINT('Origin',(0.,0.4,0.));
#18372=CARTESIAN_POINT('',(-0.652485211708638,0.,0.491682873915223));
#18373=CARTESIAN_POINT('Origin',(0.,0.,0.));
#18374=CARTESIAN_POINT('',(-0.652485211708638,0.4,-0.491682873915224));
#18375=CARTESIAN_POINT('',(-0.652485211708638,0.,-0.491682873915224));
#18376=CARTESIAN_POINT('',(-0.0995672535620054,0.4,-0.81091020589096));
#18377=CARTESIAN_POINT('Origin',(0.,0.4,0.));
#18378=CARTESIAN_POINT('',(-0.0995672535620054,0.,-0.81091020589096));
#18379=CARTESIAN_POINT('Origin',(0.,0.,0.));
#18380=CARTESIAN_POINT('',(0.652485211708638,0.4,-0.491682873915223));
#18381=CARTESIAN_POINT('',(0.652485211708638,0.,-0.491682873915223));
#18382=CARTESIAN_POINT('',(0.0995672535620056,0.4,-0.81091020589096));
#18383=CARTESIAN_POINT('',(0.0995672535620056,0.,-0.81091020589096));
#18384=CARTESIAN_POINT('Origin',(0.,0.4,0.));
#18385=CARTESIAN_POINT('Origin',(0.,0.,0.));
#18386=CARTESIAN_POINT('',(-0.752052465270644,0.4,-0.319227331975737));
#18387=CARTESIAN_POINT('',(-0.752052465270644,0.,-0.319227331975737));
#18388=CARTESIAN_POINT('',(-0.752052465270644,0.4,0.319227331975736));
#18389=CARTESIAN_POINT('',(-0.752052465270644,0.,0.319227331975736));
#18390=CARTESIAN_POINT('Origin',(0.,0.4,0.));
#18391=CARTESIAN_POINT('Origin',(0.,0.,0.));
#18392=CARTESIAN_POINT('',(0.099567253562005,0.4,0.81091020589096));
#18393=CARTESIAN_POINT('',(0.099567253562005,0.,0.81091020589096));
#18394=CARTESIAN_POINT('',(0.652485211708638,0.4,0.491682873915224));
#18395=CARTESIAN_POINT('',(0.652485211708638,0.,0.491682873915224));
#18396=CARTESIAN_POINT('Origin',(0.,0.4,0.));
#18397=CARTESIAN_POINT('Origin',(0.,0.4,0.));
#18398=CARTESIAN_POINT('',(0.0994453842185998,0.4,0.809917659739319));
#18399=CARTESIAN_POINT('',(0.0818108902278751,0.4,0.666296231596819));
#18400=CARTESIAN_POINT('',(0.65168657619859,0.4,0.491081058892072));
#18401=CARTESIAN_POINT('',(0.325843288099295,0.4,0.245540529446036));
#18402=CARTESIAN_POINT('',(0.67113967774902,0.4,0.464141716451928));
#18403=CARTESIAN_POINT('',(0.666276402361412,0.4,0.470876552061965));
#18404=CARTESIAN_POINT('',(0.689479866344547,0.4,0.436432714064271));
#18405=CARTESIAN_POINT('',(0.684894819195665,0.4,0.443359964661185));
#18406=CARTESIAN_POINT('',(0.706676729488102,0.4,0.408000000000001));
#18407=CARTESIAN_POINT('',(0.702377513702213,0.4,0.415108178516068));
#18408=CARTESIAN_POINT('',(0.722701750594521,0.4,0.378890722620143));
#18409=CARTESIAN_POINT('',(0.718695495317916,0.4,0.386168041965108));
#18410=CARTESIAN_POINT('',(0.737528356277993,0.4,0.349153152192391));
#18411=CARTESIAN_POINT('',(0.733821704857125,0.4,0.356587544799328));
#18412=CARTESIAN_POINT('',(0.751131960417191,0.4,0.318836600847248));
#18413=CARTESIAN_POINT('',(0.747731059382392,0.4,0.326415738683533));
#18414=CARTESIAN_POINT('',(0.617934908122623,0.4,0.26229780655485));
#18415=CARTESIAN_POINT('',(0.751131960417191,0.4,-0.318836600847247));
#18416=CARTESIAN_POINT('',(0.375565980208596,0.4,-0.159418300423624));
#18417=CARTESIAN_POINT('',(0.737528356277993,0.4,-0.34915315219239));
#18418=CARTESIAN_POINT('',(0.740929257312793,0.4,-0.341574014356103));
#18419=CARTESIAN_POINT('',(0.722701750594522,0.4,-0.378890722620142));
#18420=CARTESIAN_POINT('',(0.72640840201539,0.4,-0.371456330013204));
#18421=CARTESIAN_POINT('',(0.706676729488102,0.4,-0.408));
#18422=CARTESIAN_POINT('',(0.710682984764707,0.4,-0.400722680655036));
#18423=CARTESIAN_POINT('',(0.689479866344548,0.4,-0.43643271406427));
#18424=CARTESIAN_POINT('',(0.693779082130436,0.4,-0.429324535548202));
#18425=CARTESIAN_POINT('',(0.67113967774902,0.4,-0.464141716451927));
#18426=CARTESIAN_POINT('',(0.675724724897902,0.4,-0.457214465855013));
#18427=CARTESIAN_POINT('',(0.651686576198591,0.4,-0.491081058892071));
#18428=CARTESIAN_POINT('',(0.656549851586198,0.4,-0.484346223282036));
#18429=CARTESIAN_POINT('',(0.536124017894748,0.4,-0.40399842504197));
#18430=CARTESIAN_POINT('',(0.0994453842186005,0.4,-0.809917659739319));
#18431=CARTESIAN_POINT('',(0.0497226921093002,0.4,-0.404958829869659));
#18432=CARTESIAN_POINT('',(0.0663886785289726,0.4,-0.813294868644317));
#18433=CARTESIAN_POINT('',(0.0746528549513807,0.4,-0.812450566418067));
#18434=CARTESIAN_POINT('',(0.0332218842499744,0.4,-0.815323436684413));
#18435=CARTESIAN_POINT('',(0.0415135828197244,0.4,-0.814816294674389));
#18436=CARTESIAN_POINT('',(2.22044604925031E-16,0.4,-0.816));
#18437=CARTESIAN_POINT('',(0.00830547106249352,0.4,-0.815830859171103));
#18438=CARTESIAN_POINT('',(-0.033221884249974,0.4,-0.815323436684413));
#18439=CARTESIAN_POINT('',(-0.0249164131874803,0.4,-0.81549257751331));
#18440=CARTESIAN_POINT('',(-0.0663886785289722,0.4,-0.813294868644317));
#18441=CARTESIAN_POINT('',(-0.0580969799592231,0.4,-0.813802010654341));
#18442=CARTESIAN_POINT('',(-0.0994453842186002,0.4,-0.809917659739319));
#18443=CARTESIAN_POINT('',(-0.0911812077961943,0.4,-0.810761961965568));
#18444=CARTESIAN_POINT('',(-0.0818108902278754,0.4,-0.666296231596819));
#18445=CARTESIAN_POINT('',(-0.651686576198591,0.4,-0.491081058892072));
#18446=CARTESIAN_POINT('',(-0.325843288099295,0.4,-0.245540529446036));
#18447=CARTESIAN_POINT('',(-0.67113967774902,0.4,-0.464141716451927));
#18448=CARTESIAN_POINT('',(-0.666276402361412,0.4,-0.470876552061964));
#18449=CARTESIAN_POINT('',(-0.689479866344548,0.4,-0.43643271406427));
#18450=CARTESIAN_POINT('',(-0.684894819195665,0.4,-0.443359964661185));
#18451=CARTESIAN_POINT('',(-0.706676729488102,0.4,-0.408));
#18452=CARTESIAN_POINT('',(-0.702377513702213,0.4,-0.415108178516068));
#18453=CARTESIAN_POINT('',(-0.722701750594522,0.4,-0.378890722620143));
#18454=CARTESIAN_POINT('',(-0.718695495317917,0.4,-0.386168041965107));
#18455=CARTESIAN_POINT('',(-0.737528356277993,0.4,-0.34915315219239));
#18456=CARTESIAN_POINT('',(-0.733821704857125,0.4,-0.356587544799328));
#18457=CARTESIAN_POINT('',(-0.751131960417191,0.4,-0.318836600847248));
#18458=CARTESIAN_POINT('',(-0.747731059382392,0.4,-0.326415738683532));
#18459=CARTESIAN_POINT('',(-0.617934908122623,0.4,-0.26229780655485));
#18460=CARTESIAN_POINT('',(-0.751131960417191,0.4,0.318836600847247));
#18461=CARTESIAN_POINT('',(-0.375565980208596,0.4,0.159418300423624));
#18462=CARTESIAN_POINT('',(-0.737528356277993,0.4,0.34915315219239));
#18463=CARTESIAN_POINT('',(-0.740929257312793,0.4,0.341574014356103));
#18464=CARTESIAN_POINT('',(-0.722701750594522,0.4,0.378890722620142));
#18465=CARTESIAN_POINT('',(-0.72640840201539,0.4,0.371456330013204));
#18466=CARTESIAN_POINT('',(-0.706676729488102,0.4,0.408));
#18467=CARTESIAN_POINT('',(-0.710682984764707,0.4,0.400722680655036));
#18468=CARTESIAN_POINT('',(-0.689479866344548,0.4,0.43643271406427));
#18469=CARTESIAN_POINT('',(-0.693779082130436,0.4,0.429324535548202));
#18470=CARTESIAN_POINT('',(-0.671139677749021,0.4,0.464141716451927));
#18471=CARTESIAN_POINT('',(-0.675724724897902,0.4,0.457214465855013));
#18472=CARTESIAN_POINT('',(-0.651686576198591,0.4,0.491081058892071));
#18473=CARTESIAN_POINT('',(-0.656549851586198,0.4,0.484346223282036));
#18474=CARTESIAN_POINT('',(-0.536124017894748,0.4,0.40399842504197));
#18475=CARTESIAN_POINT('',(-0.0994453842186008,0.4,0.809917659739319));
#18476=CARTESIAN_POINT('',(-0.0497226921093004,0.4,0.404958829869659));
#18477=CARTESIAN_POINT('',(-0.0663886785289729,0.4,0.813294868644317));
#18478=CARTESIAN_POINT('',(-0.074652854951381,0.4,0.812450566418067));
#18479=CARTESIAN_POINT('',(-0.0332218842499747,0.4,0.815323436684413));
#18480=CARTESIAN_POINT('',(-0.0415135828197248,0.4,0.814816294674389));
#18481=CARTESIAN_POINT('',(-4.9960036108132E-16,0.4,0.816));
#18482=CARTESIAN_POINT('',(-0.00830547106249374,0.4,0.815830859171103));
#18483=CARTESIAN_POINT('',(0.0332218842499737,0.4,0.815323436684413));
#18484=CARTESIAN_POINT('',(0.0249164131874799,0.4,0.81549257751331));
#18485=CARTESIAN_POINT('',(0.0663886785289718,0.4,0.813294868644317));
#18486=CARTESIAN_POINT('',(0.0580969799592227,0.4,0.813802010654341));
#18487=CARTESIAN_POINT('',(0.091181207796194,0.4,0.810761961965568));
#18488=CARTESIAN_POINT('Origin',(1.23586981624525,0.,0.5245956131097));
#18489=CARTESIAN_POINT('',(0.751131960417191,1.,0.318836600847248));
#18490=CARTESIAN_POINT('',(0.751131960417191,0.,0.318836600847248));
#18491=CARTESIAN_POINT('',(1.23586981624525,1.,0.5245956131097));
#18492=CARTESIAN_POINT('',(1.23586981624525,1.,0.5245956131097));
#18493=CARTESIAN_POINT('',(1.23586981624525,-1.,0.5245956131097));
#18494=CARTESIAN_POINT('',(1.23586981624525,0.,0.5245956131097));
#18495=CARTESIAN_POINT('',(0.751131960417191,-1.,0.318836600847248));
#18496=CARTESIAN_POINT('',(1.23586981624525,-1.,0.5245956131097));
#18497=CARTESIAN_POINT('',(0.751131960417191,0.,0.318836600847248));
#18498=CARTESIAN_POINT('Origin',(0.751131960417191,0.,0.318836600847248));
#18499=CARTESIAN_POINT('',(0.737528356277993,1.,0.349153152192391));
#18500=CARTESIAN_POINT('',(0.737528356277993,0.,0.349153152192391));
#18501=CARTESIAN_POINT('',(0.751131960417191,1.,0.318836600847248));
#18502=CARTESIAN_POINT('Origin',(0.751131960417191,0.,0.318836600847248));
#18503=CARTESIAN_POINT('',(0.737528356277993,-1.,0.349153152192391));
#18504=CARTESIAN_POINT('',(0.751131960417191,-1.,0.318836600847248));
#18505=CARTESIAN_POINT('',(0.737528356277993,0.,0.349153152192391));
#18506=CARTESIAN_POINT('Origin',(0.737528356277993,0.,0.349153152192391));
#18507=CARTESIAN_POINT('',(0.722701750594521,1.,0.378890722620143));
#18508=CARTESIAN_POINT('',(0.722701750594521,0.,0.378890722620143));
#18509=CARTESIAN_POINT('',(0.737528356277993,1.,0.349153152192391));
#18510=CARTESIAN_POINT('Origin',(0.722701750594521,0.,0.378890722620143));
#18511=CARTESIAN_POINT('',(0.706676729488102,1.,0.408000000000001));
#18512=CARTESIAN_POINT('',(0.706676729488102,0.,0.408000000000001));
#18513=CARTESIAN_POINT('',(0.722701750594521,1.,0.378890722620143));
#18514=CARTESIAN_POINT('Origin',(0.706676729488102,0.,0.408000000000001));
#18515=CARTESIAN_POINT('',(0.689479866344547,1.,0.436432714064271));
#18516=CARTESIAN_POINT('',(0.689479866344547,0.,0.436432714064271));
#18517=CARTESIAN_POINT('',(0.706676729488102,1.,0.408000000000001));
#18518=CARTESIAN_POINT('Origin',(0.689479866344547,0.,0.436432714064271));
#18519=CARTESIAN_POINT('',(0.67113967774902,1.,0.464141716451928));
#18520=CARTESIAN_POINT('',(0.67113967774902,0.,0.464141716451928));
#18521=CARTESIAN_POINT('',(0.689479866344547,1.,0.436432714064271));
#18522=CARTESIAN_POINT('Origin',(0.67113967774902,0.,0.464141716451928));
#18523=CARTESIAN_POINT('',(0.65168657619859,1.,0.491081058892072));
#18524=CARTESIAN_POINT('',(0.65168657619859,0.,0.491081058892072));
#18525=CARTESIAN_POINT('',(0.67113967774902,1.,0.464141716451928));
#18526=CARTESIAN_POINT('Origin',(0.932067487714439,-1.,0.53812941493483));
#18527=CARTESIAN_POINT('',(1.07224803578949,-1.,0.807996850083941));
#18528=CARTESIAN_POINT('',(0.65168657619859,-1.,0.491081058892072));
#18529=CARTESIAN_POINT('',(0.65168657619859,-1.,0.491081058892072));
#18530=CARTESIAN_POINT('',(0.67113967774902,-1.,0.464141716451928));
#18531=CARTESIAN_POINT('',(0.67113967774902,-1.,0.464141716451928));
#18532=CARTESIAN_POINT('',(0.689479866344547,-1.,0.436432714064271));
#18533=CARTESIAN_POINT('',(0.689479866344547,-1.,0.436432714064271));
#18534=CARTESIAN_POINT('',(0.706676729488102,-1.,0.408000000000001));
#18535=CARTESIAN_POINT('',(0.706676729488102,-1.,0.408000000000001));
#18536=CARTESIAN_POINT('',(0.722701750594521,-1.,0.378890722620143));
#18537=CARTESIAN_POINT('',(0.722701750594521,-1.,0.378890722620143));
#18538=CARTESIAN_POINT('',(0.737528356277993,-1.,0.349153152192391));
#18539=CARTESIAN_POINT('',(1.21348721953288,-1.,0.574476742810666));
#18540=CARTESIAN_POINT('',(1.21348721953288,-1.,0.574476742810666));
#18541=CARTESIAN_POINT('',(1.1890923656228,-1.,0.623405250232603));
#18542=CARTESIAN_POINT('',(1.1890923656228,-1.,0.623405250232603));
#18543=CARTESIAN_POINT('',(1.16272570712099,-1.,0.671300000000001));
#18544=CARTESIAN_POINT('',(1.16272570712099,-1.,0.671300000000001));
#18545=CARTESIAN_POINT('',(1.13443096636543,-1.,0.718081570959179));
#18546=CARTESIAN_POINT('',(1.13443096636543,-1.,0.718081570959179));
#18547=CARTESIAN_POINT('',(1.10425506292382,-1.,0.76367238787789));
#18548=CARTESIAN_POINT('',(1.10425506292382,-1.,0.76367238787789));
#18549=CARTESIAN_POINT('',(1.07224803578949,-1.,0.807996850083941));
#18550=CARTESIAN_POINT('Origin',(0.67113967774902,0.,0.464141716451928));
#18551=CARTESIAN_POINT('',(0.67113967774902,0.,0.464141716451928));
#18552=CARTESIAN_POINT('',(0.65168657619859,0.,0.491081058892072));
#18553=CARTESIAN_POINT('Origin',(0.689479866344547,0.,0.436432714064271));
#18554=CARTESIAN_POINT('',(0.689479866344547,0.,0.436432714064271));
#18555=CARTESIAN_POINT('Origin',(0.706676729488102,0.,0.408000000000001));
#18556=CARTESIAN_POINT('',(0.706676729488102,0.,0.408000000000001));
#18557=CARTESIAN_POINT('Origin',(0.722701750594521,0.,0.378890722620143));
#18558=CARTESIAN_POINT('',(0.722701750594521,0.,0.378890722620143));
#18559=CARTESIAN_POINT('Origin',(0.737528356277993,0.,0.349153152192391));
#18560=CARTESIAN_POINT('Origin',(1.21348721953288,0.,0.574476742810666));
#18561=CARTESIAN_POINT('',(1.21348721953288,1.,0.574476742810666));
#18562=CARTESIAN_POINT('',(1.21348721953288,1.,0.574476742810666));
#18563=CARTESIAN_POINT('',(1.21348721953288,0.,0.574476742810666));
#18564=CARTESIAN_POINT('Origin',(1.1890923656228,0.,0.623405250232603));
#18565=CARTESIAN_POINT('',(1.1890923656228,1.,0.623405250232603));
#18566=CARTESIAN_POINT('',(1.1890923656228,1.,0.623405250232603));
#18567=CARTESIAN_POINT('',(1.1890923656228,0.,0.623405250232603));
#18568=CARTESIAN_POINT('Origin',(1.16272570712099,0.,0.671300000000001));
#18569=CARTESIAN_POINT('',(1.16272570712099,1.,0.671300000000001));
#18570=CARTESIAN_POINT('',(1.16272570712099,1.,0.671300000000001));
#18571=CARTESIAN_POINT('',(1.16272570712099,0.,0.671300000000001));
#18572=CARTESIAN_POINT('Origin',(1.13443096636543,0.,0.718081570959179));
#18573=CARTESIAN_POINT('',(1.13443096636543,1.,0.718081570959179));
#18574=CARTESIAN_POINT('',(1.13443096636543,1.,0.718081570959179));
#18575=CARTESIAN_POINT('',(1.13443096636543,0.,0.718081570959179));
#18576=CARTESIAN_POINT('Origin',(1.10425506292382,0.,0.76367238787789));
#18577=CARTESIAN_POINT('',(1.10425506292382,1.,0.76367238787789));
#18578=CARTESIAN_POINT('',(1.10425506292382,1.,0.76367238787789));
#18579=CARTESIAN_POINT('',(1.10425506292382,0.,0.76367238787789));
#18580=CARTESIAN_POINT('Origin',(1.07224803578949,0.,0.807996850083941));
#18581=CARTESIAN_POINT('',(1.07224803578949,1.,0.807996850083941));
#18582=CARTESIAN_POINT('',(1.07224803578949,1.,0.807996850083941));
#18583=CARTESIAN_POINT('',(1.07224803578949,0.,0.807996850083941));
#18584=CARTESIAN_POINT('Origin',(0.65168657619859,0.,0.491081058892072));
#18585=CARTESIAN_POINT('',(0.65168657619859,1.,0.491081058892072));
#18586=CARTESIAN_POINT('Origin',(0.932067487714439,1.,0.53812941493483));
#18587=CARTESIAN_POINT('Origin',(-1.0722480357895,0.,0.80799685008394));
#18588=CARTESIAN_POINT('',(-0.651686576198591,1.,0.491081058892071));
#18589=CARTESIAN_POINT('',(-0.651686576198591,0.,0.491081058892071));
#18590=CARTESIAN_POINT('',(-1.0722480357895,1.,0.80799685008394));
#18591=CARTESIAN_POINT('',(-1.0722480357895,1.,0.80799685008394));
#18592=CARTESIAN_POINT('',(-1.0722480357895,-1.,0.80799685008394));
#18593=CARTESIAN_POINT('',(-1.0722480357895,0.,0.80799685008394));
#18594=CARTESIAN_POINT('',(-0.651686576198591,-1.,0.491081058892071));
#18595=CARTESIAN_POINT('',(-1.0722480357895,-1.,0.80799685008394));
#18596=CARTESIAN_POINT('',(-0.651686576198591,0.,0.491081058892071));
#18597=CARTESIAN_POINT('Origin',(-0.651686576198591,0.,0.491081058892071));
#18598=CARTESIAN_POINT('',(-0.671139677749021,1.,0.464141716451927));
#18599=CARTESIAN_POINT('',(-0.671139677749021,0.,0.464141716451927));
#18600=CARTESIAN_POINT('',(-0.651686576198591,1.,0.491081058892071));
#18601=CARTESIAN_POINT('Origin',(-0.651686576198591,0.,0.491081058892071));
#18602=CARTESIAN_POINT('',(-0.671139677749021,-1.,0.464141716451927));
#18603=CARTESIAN_POINT('',(-0.651686576198591,-1.,0.491081058892071));
#18604=CARTESIAN_POINT('',(-0.671139677749021,0.,0.464141716451927));
#18605=CARTESIAN_POINT('Origin',(-0.671139677749021,0.,0.464141716451927));
#18606=CARTESIAN_POINT('',(-0.689479866344548,1.,0.43643271406427));
#18607=CARTESIAN_POINT('',(-0.689479866344548,0.,0.43643271406427));
#18608=CARTESIAN_POINT('',(-0.671139677749021,1.,0.464141716451927));
#18609=CARTESIAN_POINT('Origin',(-0.689479866344548,0.,0.43643271406427));
#18610=CARTESIAN_POINT('',(-0.706676729488102,1.,0.408));
#18611=CARTESIAN_POINT('',(-0.706676729488102,0.,0.408));
#18612=CARTESIAN_POINT('',(-0.689479866344548,1.,0.43643271406427));
#18613=CARTESIAN_POINT('Origin',(-0.706676729488102,0.,0.408));
#18614=CARTESIAN_POINT('',(-0.722701750594522,1.,0.378890722620142));
#18615=CARTESIAN_POINT('',(-0.722701750594522,0.,0.378890722620142));
#18616=CARTESIAN_POINT('',(-0.706676729488102,1.,0.408));
#18617=CARTESIAN_POINT('Origin',(-0.722701750594522,0.,0.378890722620142));
#18618=CARTESIAN_POINT('',(-0.737528356277993,1.,0.34915315219239));
#18619=CARTESIAN_POINT('',(-0.737528356277993,0.,0.34915315219239));
#18620=CARTESIAN_POINT('',(-0.722701750594522,1.,0.378890722620142));
#18621=CARTESIAN_POINT('Origin',(-0.737528356277993,0.,0.34915315219239));
#18622=CARTESIAN_POINT('',(-0.751131960417191,1.,0.318836600847247));
#18623=CARTESIAN_POINT('',(-0.751131960417191,0.,0.318836600847247));
#18624=CARTESIAN_POINT('',(-0.737528356277993,1.,0.34915315219239));
#18625=CARTESIAN_POINT('Origin',(-0.932067487714439,-1.,0.538129414934829));
#18626=CARTESIAN_POINT('',(-1.23586981624525,-1.,0.524595613109699));
#18627=CARTESIAN_POINT('',(-0.751131960417191,-1.,0.318836600847247));
#18628=CARTESIAN_POINT('',(-0.751131960417191,-1.,0.318836600847247));
#18629=CARTESIAN_POINT('',(-0.737528356277993,-1.,0.34915315219239));
#18630=CARTESIAN_POINT('',(-0.737528356277993,-1.,0.34915315219239));
#18631=CARTESIAN_POINT('',(-0.722701750594522,-1.,0.378890722620142));
#18632=CARTESIAN_POINT('',(-0.722701750594522,-1.,0.378890722620142));
#18633=CARTESIAN_POINT('',(-0.706676729488102,-1.,0.408));
#18634=CARTESIAN_POINT('',(-0.706676729488102,-1.,0.408));
#18635=CARTESIAN_POINT('',(-0.689479866344548,-1.,0.43643271406427));
#18636=CARTESIAN_POINT('',(-0.689479866344548,-1.,0.43643271406427));
#18637=CARTESIAN_POINT('',(-0.671139677749021,-1.,0.464141716451927));
#18638=CARTESIAN_POINT('',(-1.10425506292382,-1.,0.763672387877888));
#18639=CARTESIAN_POINT('',(-1.10425506292382,-1.,0.763672387877888));
#18640=CARTESIAN_POINT('',(-1.13443096636543,-1.,0.718081570959177));
#18641=CARTESIAN_POINT('',(-1.13443096636543,-1.,0.718081570959177));
#18642=CARTESIAN_POINT('',(-1.16272570712099,-1.,0.6713));
#18643=CARTESIAN_POINT('',(-1.16272570712099,-1.,0.6713));
#18644=CARTESIAN_POINT('',(-1.1890923656228,-1.,0.623405250232602));
#18645=CARTESIAN_POINT('',(-1.1890923656228,-1.,0.623405250232602));
#18646=CARTESIAN_POINT('',(-1.21348721953288,-1.,0.574476742810665));
#18647=CARTESIAN_POINT('',(-1.21348721953288,-1.,0.574476742810665));
#18648=CARTESIAN_POINT('',(-1.23586981624525,-1.,0.524595613109699));
#18649=CARTESIAN_POINT('Origin',(-0.737528356277993,0.,0.34915315219239));
#18650=CARTESIAN_POINT('',(-0.737528356277993,0.,0.34915315219239));
#18651=CARTESIAN_POINT('',(-0.751131960417191,0.,0.318836600847247));
#18652=CARTESIAN_POINT('Origin',(-0.722701750594522,0.,0.378890722620142));
#18653=CARTESIAN_POINT('',(-0.722701750594522,0.,0.378890722620142));
#18654=CARTESIAN_POINT('Origin',(-0.706676729488102,0.,0.408));
#18655=CARTESIAN_POINT('',(-0.706676729488102,0.,0.408));
#18656=CARTESIAN_POINT('Origin',(-0.689479866344548,0.,0.43643271406427));
#18657=CARTESIAN_POINT('',(-0.689479866344548,0.,0.43643271406427));
#18658=CARTESIAN_POINT('Origin',(-0.671139677749021,0.,0.464141716451927));
#18659=CARTESIAN_POINT('Origin',(-1.10425506292382,0.,0.763672387877888));
#18660=CARTESIAN_POINT('',(-1.10425506292382,1.,0.763672387877888));
#18661=CARTESIAN_POINT('',(-1.10425506292382,1.,0.763672387877888));
#18662=CARTESIAN_POINT('',(-1.10425506292382,0.,0.763672387877888));
#18663=CARTESIAN_POINT('Origin',(-1.13443096636543,0.,0.718081570959177));
#18664=CARTESIAN_POINT('',(-1.13443096636543,1.,0.718081570959177));
#18665=CARTESIAN_POINT('',(-1.13443096636543,1.,0.718081570959177));
#18666=CARTESIAN_POINT('',(-1.13443096636543,0.,0.718081570959177));
#18667=CARTESIAN_POINT('Origin',(-1.16272570712099,0.,0.6713));
#18668=CARTESIAN_POINT('',(-1.16272570712099,1.,0.6713));
#18669=CARTESIAN_POINT('',(-1.16272570712099,1.,0.6713));
#18670=CARTESIAN_POINT('',(-1.16272570712099,0.,0.6713));
#18671=CARTESIAN_POINT('Origin',(-1.1890923656228,0.,0.623405250232602));
#18672=CARTESIAN_POINT('',(-1.1890923656228,1.,0.623405250232602));
#18673=CARTESIAN_POINT('',(-1.1890923656228,1.,0.623405250232602));
#18674=CARTESIAN_POINT('',(-1.1890923656228,0.,0.623405250232602));
#18675=CARTESIAN_POINT('Origin',(-1.21348721953288,0.,0.574476742810665));
#18676=CARTESIAN_POINT('',(-1.21348721953288,1.,0.574476742810665));
#18677=CARTESIAN_POINT('',(-1.21348721953288,1.,0.574476742810665));
#18678=CARTESIAN_POINT('',(-1.21348721953288,0.,0.574476742810665));
#18679=CARTESIAN_POINT('Origin',(-1.23586981624525,0.,0.524595613109699));
#18680=CARTESIAN_POINT('',(-1.23586981624525,1.,0.524595613109699));
#18681=CARTESIAN_POINT('',(-1.23586981624525,1.,0.524595613109699));
#18682=CARTESIAN_POINT('',(-1.23586981624525,0.,0.524595613109699));
#18683=CARTESIAN_POINT('Origin',(-0.751131960417191,0.,0.318836600847247));
#18684=CARTESIAN_POINT('',(-0.751131960417191,1.,0.318836600847247));
#18685=CARTESIAN_POINT('Origin',(-0.932067487714439,1.,0.538129414934829));
#18686=CARTESIAN_POINT('Origin',(-0.163621780455751,0.,-1.33259246319364));
#18687=CARTESIAN_POINT('',(-0.0994453842186002,1.,-0.809917659739319));
#18688=CARTESIAN_POINT('',(-0.0994453842186002,0.,-0.809917659739319));
#18689=CARTESIAN_POINT('',(-0.163621780455751,1.,-1.33259246319364));
#18690=CARTESIAN_POINT('',(-0.163621780455751,1.,-1.33259246319364));
#18691=CARTESIAN_POINT('',(-0.163621780455751,-1.,-1.33259246319364));
#18692=CARTESIAN_POINT('',(-0.163621780455751,0.,-1.33259246319364));
#18693=CARTESIAN_POINT('',(-0.0994453842186002,-1.,-0.809917659739319));
#18694=CARTESIAN_POINT('',(-0.163621780455751,-1.,-1.33259246319364));
#18695=CARTESIAN_POINT('',(-0.0994453842186002,0.,-0.809917659739319));
#18696=CARTESIAN_POINT('Origin',(-0.0994453842186002,0.,-0.809917659739319));
#18697=CARTESIAN_POINT('',(-0.0663886785289722,1.,-0.813294868644317));
#18698=CARTESIAN_POINT('',(-0.0663886785289722,0.,-0.813294868644317));
#18699=CARTESIAN_POINT('',(-0.0994453842186002,1.,-0.809917659739319));
#18700=CARTESIAN_POINT('Origin',(-0.0994453842186002,0.,-0.809917659739319));
#18701=CARTESIAN_POINT('',(-0.0663886785289722,-1.,-0.813294868644317));
#18702=CARTESIAN_POINT('',(-0.0994453842186002,-1.,-0.809917659739319));
#18703=CARTESIAN_POINT('',(-0.0663886785289722,0.,-0.813294868644317));
#18704=CARTESIAN_POINT('Origin',(-0.0663886785289722,0.,-0.813294868644317));
#18705=CARTESIAN_POINT('',(-0.033221884249974,1.,-0.815323436684413));
#18706=CARTESIAN_POINT('',(-0.033221884249974,0.,-0.815323436684413));
#18707=CARTESIAN_POINT('',(-0.0663886785289722,1.,-0.813294868644317));
#18708=CARTESIAN_POINT('Origin',(-0.033221884249974,0.,-0.815323436684413));
#18709=CARTESIAN_POINT('',(2.22044604925031E-16,1.,-0.816));
#18710=CARTESIAN_POINT('',(2.22044604925031E-16,0.,-0.816));
#18711=CARTESIAN_POINT('',(-0.033221884249974,1.,-0.815323436684413));
#18712=CARTESIAN_POINT('Origin',(2.22044604925031E-16,0.,-0.816));
#18713=CARTESIAN_POINT('',(0.0332218842499744,1.,-0.815323436684413));
#18714=CARTESIAN_POINT('',(0.0332218842499744,0.,-0.815323436684413));
#18715=CARTESIAN_POINT('',(2.22044604925031E-16,1.,-0.816));
#18716=CARTESIAN_POINT('Origin',(0.0332218842499744,0.,-0.815323436684413));
#18717=CARTESIAN_POINT('',(0.0663886785289726,1.,-0.813294868644317));
#18718=CARTESIAN_POINT('',(0.0663886785289726,0.,-0.813294868644317));
#18719=CARTESIAN_POINT('',(0.0332218842499744,1.,-0.815323436684413));
#18720=CARTESIAN_POINT('Origin',(0.0663886785289726,0.,-0.813294868644317));
#18721=CARTESIAN_POINT('',(0.0994453842186005,1.,-0.809917659739319));
#18722=CARTESIAN_POINT('',(0.0994453842186005,0.,-0.809917659739319));
#18723=CARTESIAN_POINT('',(0.0663886785289726,1.,-0.813294868644317));
#18724=CARTESIAN_POINT('Origin',(2.22044604925031E-16,-1.,-1.07625882986966));
#18725=CARTESIAN_POINT('',(0.163621780455751,-1.,-1.33259246319364));
#18726=CARTESIAN_POINT('',(0.0994453842186005,-1.,-0.809917659739319));
#18727=CARTESIAN_POINT('',(0.0994453842186005,-1.,-0.809917659739319));
#18728=CARTESIAN_POINT('',(0.0663886785289726,-1.,-0.813294868644317));
#18729=CARTESIAN_POINT('',(0.0663886785289726,-1.,-0.813294868644317));
#18730=CARTESIAN_POINT('',(0.0332218842499744,-1.,-0.815323436684413));
#18731=CARTESIAN_POINT('',(0.0332218842499744,-1.,-0.815323436684413));
#18732=CARTESIAN_POINT('',(2.22044604925031E-16,-1.,-0.816));
#18733=CARTESIAN_POINT('',(2.22044604925031E-16,-1.,-0.816));
#18734=CARTESIAN_POINT('',(-0.033221884249974,-1.,-0.815323436684413));
#18735=CARTESIAN_POINT('',(-0.033221884249974,-1.,-0.815323436684413));
#18736=CARTESIAN_POINT('',(-0.0663886785289722,-1.,-0.813294868644317));
#18737=CARTESIAN_POINT('',(-0.109232156609066,-1.,-1.33814913068855));
#18738=CARTESIAN_POINT('',(-0.109232156609066,-1.,-1.33814913068855));
#18739=CARTESIAN_POINT('',(-0.0546613992573715,-1.,-1.34148682119178));
#18740=CARTESIAN_POINT('',(-0.0546613992573715,-1.,-1.34148682119178));
#18741=CARTESIAN_POINT('',(2.22044604925031E-16,-1.,-1.3426));
#18742=CARTESIAN_POINT('',(2.22044604925031E-16,-1.,-1.3426));
#18743=CARTESIAN_POINT('',(0.054661399257372,-1.,-1.34148682119178));
#18744=CARTESIAN_POINT('',(0.054661399257372,-1.,-1.34148682119178));
#18745=CARTESIAN_POINT('',(0.109232156609067,-1.,-1.33814913068855));
#18746=CARTESIAN_POINT('',(0.109232156609067,-1.,-1.33814913068855));
#18747=CARTESIAN_POINT('',(0.163621780455751,-1.,-1.33259246319364));
#18748=CARTESIAN_POINT('Origin',(0.0663886785289726,0.,-0.813294868644317));
#18749=CARTESIAN_POINT('',(0.0663886785289726,0.,-0.813294868644317));
#18750=CARTESIAN_POINT('',(0.0994453842186005,0.,-0.809917659739319));
#18751=CARTESIAN_POINT('Origin',(0.0332218842499744,0.,-0.815323436684413));
#18752=CARTESIAN_POINT('',(0.0332218842499744,0.,-0.815323436684413));
#18753=CARTESIAN_POINT('Origin',(2.22044604925031E-16,0.,-0.816));
#18754=CARTESIAN_POINT('',(2.22044604925031E-16,0.,-0.816));
#18755=CARTESIAN_POINT('Origin',(-0.033221884249974,0.,-0.815323436684413));
#18756=CARTESIAN_POINT('',(-0.033221884249974,0.,-0.815323436684413));
#18757=CARTESIAN_POINT('Origin',(-0.0663886785289722,0.,-0.813294868644317));
#18758=CARTESIAN_POINT('Origin',(-0.109232156609066,0.,-1.33814913068855));
#18759=CARTESIAN_POINT('',(-0.109232156609066,1.,-1.33814913068855));
#18760=CARTESIAN_POINT('',(-0.109232156609066,1.,-1.33814913068855));
#18761=CARTESIAN_POINT('',(-0.109232156609066,0.,-1.33814913068855));
#18762=CARTESIAN_POINT('Origin',(-0.0546613992573715,0.,-1.34148682119178));
#18763=CARTESIAN_POINT('',(-0.0546613992573715,1.,-1.34148682119178));
#18764=CARTESIAN_POINT('',(-0.0546613992573715,1.,-1.34148682119178));
#18765=CARTESIAN_POINT('',(-0.0546613992573715,0.,-1.34148682119178));
#18766=CARTESIAN_POINT('Origin',(2.22044604925031E-16,0.,-1.3426));
#18767=CARTESIAN_POINT('',(2.22044604925031E-16,1.,-1.3426));
#18768=CARTESIAN_POINT('',(2.22044604925031E-16,1.,-1.3426));
#18769=CARTESIAN_POINT('',(2.22044604925031E-16,0.,-1.3426));
#18770=CARTESIAN_POINT('Origin',(0.054661399257372,0.,-1.34148682119178));
#18771=CARTESIAN_POINT('',(0.054661399257372,1.,-1.34148682119178));
#18772=CARTESIAN_POINT('',(0.054661399257372,1.,-1.34148682119178));
#18773=CARTESIAN_POINT('',(0.054661399257372,0.,-1.34148682119178));
#18774=CARTESIAN_POINT('Origin',(0.109232156609067,0.,-1.33814913068855));
#18775=CARTESIAN_POINT('',(0.109232156609067,1.,-1.33814913068855));
#18776=CARTESIAN_POINT('',(0.109232156609067,1.,-1.33814913068855));
#18777=CARTESIAN_POINT('',(0.109232156609067,0.,-1.33814913068855));
#18778=CARTESIAN_POINT('Origin',(0.163621780455751,0.,-1.33259246319364));
#18779=CARTESIAN_POINT('',(0.163621780455751,1.,-1.33259246319364));
#18780=CARTESIAN_POINT('',(0.163621780455751,1.,-1.33259246319364));
#18781=CARTESIAN_POINT('',(0.163621780455751,0.,-1.33259246319364));
#18782=CARTESIAN_POINT('Origin',(0.0994453842186005,0.,-0.809917659739319));
#18783=CARTESIAN_POINT('',(0.0994453842186005,1.,-0.809917659739319));
#18784=CARTESIAN_POINT('Origin',(2.22044604925031E-16,1.,-1.07625882986966));
#18785=CARTESIAN_POINT('Origin',(1.0722480357895,0.,-0.80799685008394));
#18786=CARTESIAN_POINT('',(0.651686576198591,1.,-0.491081058892071));
#18787=CARTESIAN_POINT('',(0.651686576198591,0.,-0.491081058892071));
#18788=CARTESIAN_POINT('',(1.0722480357895,1.,-0.80799685008394));
#18789=CARTESIAN_POINT('',(1.0722480357895,1.,-0.80799685008394));
#18790=CARTESIAN_POINT('',(1.0722480357895,-1.,-0.80799685008394));
#18791=CARTESIAN_POINT('',(1.0722480357895,0.,-0.80799685008394));
#18792=CARTESIAN_POINT('',(0.651686576198591,-1.,-0.491081058892071));
#18793=CARTESIAN_POINT('',(1.0722480357895,-1.,-0.80799685008394));
#18794=CARTESIAN_POINT('',(0.651686576198591,0.,-0.491081058892071));
#18795=CARTESIAN_POINT('Origin',(0.651686576198591,0.,-0.491081058892071));
#18796=CARTESIAN_POINT('',(0.67113967774902,1.,-0.464141716451927));
#18797=CARTESIAN_POINT('',(0.67113967774902,0.,-0.464141716451927));
#18798=CARTESIAN_POINT('',(0.651686576198591,1.,-0.491081058892071));
#18799=CARTESIAN_POINT('Origin',(0.651686576198591,0.,-0.491081058892071));
#18800=CARTESIAN_POINT('',(0.67113967774902,-1.,-0.464141716451927));
#18801=CARTESIAN_POINT('',(0.651686576198591,-1.,-0.491081058892071));
#18802=CARTESIAN_POINT('',(0.67113967774902,0.,-0.464141716451927));
#18803=CARTESIAN_POINT('Origin',(0.67113967774902,0.,-0.464141716451927));
#18804=CARTESIAN_POINT('',(0.689479866344548,1.,-0.43643271406427));
#18805=CARTESIAN_POINT('',(0.689479866344548,0.,-0.43643271406427));
#18806=CARTESIAN_POINT('',(0.67113967774902,1.,-0.464141716451927));
#18807=CARTESIAN_POINT('Origin',(0.689479866344548,0.,-0.43643271406427));
#18808=CARTESIAN_POINT('',(0.706676729488102,1.,-0.408));
#18809=CARTESIAN_POINT('',(0.706676729488102,0.,-0.408));
#18810=CARTESIAN_POINT('',(0.689479866344548,1.,-0.43643271406427));
#18811=CARTESIAN_POINT('Origin',(0.706676729488102,0.,-0.408));
#18812=CARTESIAN_POINT('',(0.722701750594522,1.,-0.378890722620142));
#18813=CARTESIAN_POINT('',(0.722701750594522,0.,-0.378890722620142));
#18814=CARTESIAN_POINT('',(0.706676729488102,1.,-0.408));
#18815=CARTESIAN_POINT('Origin',(0.722701750594522,0.,-0.378890722620142));
#18816=CARTESIAN_POINT('',(0.737528356277993,1.,-0.34915315219239));
#18817=CARTESIAN_POINT('',(0.737528356277993,0.,-0.34915315219239));
#18818=CARTESIAN_POINT('',(0.722701750594522,1.,-0.378890722620142));
#18819=CARTESIAN_POINT('Origin',(0.737528356277993,0.,-0.34915315219239));
#18820=CARTESIAN_POINT('',(0.751131960417191,1.,-0.318836600847247));
#18821=CARTESIAN_POINT('',(0.751131960417191,0.,-0.318836600847247));
#18822=CARTESIAN_POINT('',(0.737528356277993,1.,-0.34915315219239));
#18823=CARTESIAN_POINT('Origin',(0.932067487714439,-1.,-0.53812941493483));
#18824=CARTESIAN_POINT('',(1.23586981624525,-1.,-0.524595613109699));
#18825=CARTESIAN_POINT('',(0.751131960417191,-1.,-0.318836600847247));
#18826=CARTESIAN_POINT('',(0.751131960417191,-1.,-0.318836600847247));
#18827=CARTESIAN_POINT('',(0.737528356277993,-1.,-0.34915315219239));
#18828=CARTESIAN_POINT('',(0.737528356277993,-1.,-0.34915315219239));
#18829=CARTESIAN_POINT('',(0.722701750594522,-1.,-0.378890722620142));
#18830=CARTESIAN_POINT('',(0.722701750594522,-1.,-0.378890722620142));
#18831=CARTESIAN_POINT('',(0.706676729488102,-1.,-0.408));
#18832=CARTESIAN_POINT('',(0.706676729488102,-1.,-0.408));
#18833=CARTESIAN_POINT('',(0.689479866344548,-1.,-0.43643271406427));
#18834=CARTESIAN_POINT('',(0.689479866344548,-1.,-0.43643271406427));
#18835=CARTESIAN_POINT('',(0.67113967774902,-1.,-0.464141716451927));
#18836=CARTESIAN_POINT('',(1.10425506292382,-1.,-0.763672387877889));
#18837=CARTESIAN_POINT('',(1.10425506292382,-1.,-0.763672387877889));
#18838=CARTESIAN_POINT('',(1.13443096636543,-1.,-0.718081570959178));
#18839=CARTESIAN_POINT('',(1.13443096636543,-1.,-0.718081570959177));
#18840=CARTESIAN_POINT('',(1.16272570712099,-1.,-0.6713));
#18841=CARTESIAN_POINT('',(1.16272570712099,-1.,-0.6713));
#18842=CARTESIAN_POINT('',(1.1890923656228,-1.,-0.623405250232602));
#18843=CARTESIAN_POINT('',(1.1890923656228,-1.,-0.623405250232602));
#18844=CARTESIAN_POINT('',(1.21348721953288,-1.,-0.574476742810665));
#18845=CARTESIAN_POINT('',(1.21348721953288,-1.,-0.574476742810665));
#18846=CARTESIAN_POINT('',(1.23586981624525,-1.,-0.524595613109699));
#18847=CARTESIAN_POINT('Origin',(0.737528356277993,0.,-0.34915315219239));
#18848=CARTESIAN_POINT('',(0.737528356277993,0.,-0.34915315219239));
#18849=CARTESIAN_POINT('',(0.751131960417191,0.,-0.318836600847247));
#18850=CARTESIAN_POINT('Origin',(0.722701750594522,0.,-0.378890722620142));
#18851=CARTESIAN_POINT('',(0.722701750594522,0.,-0.378890722620142));
#18852=CARTESIAN_POINT('Origin',(0.706676729488102,0.,-0.408));
#18853=CARTESIAN_POINT('',(0.706676729488102,0.,-0.408));
#18854=CARTESIAN_POINT('Origin',(0.689479866344548,0.,-0.43643271406427));
#18855=CARTESIAN_POINT('',(0.689479866344548,0.,-0.43643271406427));
#18856=CARTESIAN_POINT('Origin',(0.67113967774902,0.,-0.464141716451927));
#18857=CARTESIAN_POINT('Origin',(1.10425506292382,0.,-0.763672387877889));
#18858=CARTESIAN_POINT('',(1.10425506292382,1.,-0.763672387877889));
#18859=CARTESIAN_POINT('',(1.10425506292382,1.,-0.763672387877889));
#18860=CARTESIAN_POINT('',(1.10425506292382,0.,-0.763672387877889));
#18861=CARTESIAN_POINT('Origin',(1.13443096636543,0.,-0.718081570959177));
#18862=CARTESIAN_POINT('',(1.13443096636543,1.,-0.718081570959178));
#18863=CARTESIAN_POINT('',(1.13443096636543,1.,-0.718081570959177));
#18864=CARTESIAN_POINT('',(1.13443096636543,0.,-0.718081570959177));
#18865=CARTESIAN_POINT('Origin',(1.16272570712099,0.,-0.6713));
#18866=CARTESIAN_POINT('',(1.16272570712099,1.,-0.6713));
#18867=CARTESIAN_POINT('',(1.16272570712099,1.,-0.6713));
#18868=CARTESIAN_POINT('',(1.16272570712099,0.,-0.6713));
#18869=CARTESIAN_POINT('Origin',(1.1890923656228,0.,-0.623405250232602));
#18870=CARTESIAN_POINT('',(1.1890923656228,1.,-0.623405250232602));
#18871=CARTESIAN_POINT('',(1.1890923656228,1.,-0.623405250232602));
#18872=CARTESIAN_POINT('',(1.1890923656228,0.,-0.623405250232602));
#18873=CARTESIAN_POINT('Origin',(1.21348721953288,0.,-0.574476742810665));
#18874=CARTESIAN_POINT('',(1.21348721953288,1.,-0.574476742810665));
#18875=CARTESIAN_POINT('',(1.21348721953288,1.,-0.574476742810665));
#18876=CARTESIAN_POINT('',(1.21348721953288,0.,-0.574476742810665));
#18877=CARTESIAN_POINT('Origin',(1.23586981624525,0.,-0.524595613109699));
#18878=CARTESIAN_POINT('',(1.23586981624525,1.,-0.524595613109699));
#18879=CARTESIAN_POINT('',(1.23586981624525,1.,-0.524595613109699));
#18880=CARTESIAN_POINT('',(1.23586981624525,0.,-0.524595613109699));
#18881=CARTESIAN_POINT('Origin',(0.751131960417191,0.,-0.318836600847247));
#18882=CARTESIAN_POINT('',(0.751131960417191,1.,-0.318836600847247));
#18883=CARTESIAN_POINT('Origin',(0.932067487714439,1.,-0.53812941493483));
#18884=CARTESIAN_POINT('Origin',(-1.23586981624525,0.,-0.524595613109699));
#18885=CARTESIAN_POINT('',(-0.751131960417191,1.,-0.318836600847248));
#18886=CARTESIAN_POINT('',(-0.751131960417191,0.,-0.318836600847248));
#18887=CARTESIAN_POINT('',(-1.23586981624525,1.,-0.524595613109699));
#18888=CARTESIAN_POINT('',(-1.23586981624525,1.,-0.524595613109699));
#18889=CARTESIAN_POINT('',(-1.23586981624525,-1.,-0.524595613109699));
#18890=CARTESIAN_POINT('',(-1.23586981624525,0.,-0.524595613109699));
#18891=CARTESIAN_POINT('',(-0.751131960417191,-1.,-0.318836600847248));
#18892=CARTESIAN_POINT('',(-1.23586981624525,-1.,-0.524595613109699));
#18893=CARTESIAN_POINT('',(-0.751131960417191,0.,-0.318836600847248));
#18894=CARTESIAN_POINT('Origin',(-0.751131960417191,0.,-0.318836600847248));
#18895=CARTESIAN_POINT('',(-0.737528356277993,1.,-0.34915315219239));
#18896=CARTESIAN_POINT('',(-0.737528356277993,0.,-0.34915315219239));
#18897=CARTESIAN_POINT('',(-0.751131960417191,1.,-0.318836600847248));
#18898=CARTESIAN_POINT('Origin',(-0.751131960417191,0.,-0.318836600847248));
#18899=CARTESIAN_POINT('',(-0.737528356277993,-1.,-0.34915315219239));
#18900=CARTESIAN_POINT('',(-0.751131960417191,-1.,-0.318836600847248));
#18901=CARTESIAN_POINT('',(-0.737528356277993,0.,-0.34915315219239));
#18902=CARTESIAN_POINT('Origin',(-0.737528356277993,0.,-0.34915315219239));
#18903=CARTESIAN_POINT('',(-0.722701750594522,1.,-0.378890722620143));
#18904=CARTESIAN_POINT('',(-0.722701750594522,0.,-0.378890722620143));
#18905=CARTESIAN_POINT('',(-0.737528356277993,1.,-0.34915315219239));
#18906=CARTESIAN_POINT('Origin',(-0.722701750594522,0.,-0.378890722620143));
#18907=CARTESIAN_POINT('',(-0.706676729488102,1.,-0.408));
#18908=CARTESIAN_POINT('',(-0.706676729488102,0.,-0.408));
#18909=CARTESIAN_POINT('',(-0.722701750594522,1.,-0.378890722620143));
#18910=CARTESIAN_POINT('Origin',(-0.706676729488102,0.,-0.408));
#18911=CARTESIAN_POINT('',(-0.689479866344548,1.,-0.43643271406427));
#18912=CARTESIAN_POINT('',(-0.689479866344548,0.,-0.43643271406427));
#18913=CARTESIAN_POINT('',(-0.706676729488102,1.,-0.408));
#18914=CARTESIAN_POINT('Origin',(-0.689479866344548,0.,-0.43643271406427));
#18915=CARTESIAN_POINT('',(-0.67113967774902,1.,-0.464141716451927));
#18916=CARTESIAN_POINT('',(-0.67113967774902,0.,-0.464141716451927));
#18917=CARTESIAN_POINT('',(-0.689479866344548,1.,-0.43643271406427));
#18918=CARTESIAN_POINT('Origin',(-0.67113967774902,0.,-0.464141716451927));
#18919=CARTESIAN_POINT('',(-0.651686576198591,1.,-0.491081058892072));
#18920=CARTESIAN_POINT('',(-0.651686576198591,0.,-0.491081058892072));
#18921=CARTESIAN_POINT('',(-0.67113967774902,1.,-0.464141716451927));
#18922=CARTESIAN_POINT('Origin',(-0.932067487714439,-1.,-0.53812941493483));
#18923=CARTESIAN_POINT('',(-1.0722480357895,-1.,-0.80799685008394));
#18924=CARTESIAN_POINT('',(-0.651686576198591,-1.,-0.491081058892072));
#18925=CARTESIAN_POINT('',(-0.651686576198591,-1.,-0.491081058892072));
#18926=CARTESIAN_POINT('',(-0.67113967774902,-1.,-0.464141716451927));
#18927=CARTESIAN_POINT('',(-0.67113967774902,-1.,-0.464141716451927));
#18928=CARTESIAN_POINT('',(-0.689479866344548,-1.,-0.43643271406427));
#18929=CARTESIAN_POINT('',(-0.689479866344548,-1.,-0.43643271406427));
#18930=CARTESIAN_POINT('',(-0.706676729488102,-1.,-0.408));
#18931=CARTESIAN_POINT('',(-0.706676729488102,-1.,-0.408));
#18932=CARTESIAN_POINT('',(-0.722701750594522,-1.,-0.378890722620143));
#18933=CARTESIAN_POINT('',(-0.722701750594522,-1.,-0.378890722620143));
#18934=CARTESIAN_POINT('',(-0.737528356277993,-1.,-0.34915315219239));
#18935=CARTESIAN_POINT('',(-1.21348721953288,-1.,-0.574476742810665));
#18936=CARTESIAN_POINT('',(-1.21348721953288,-1.,-0.574476742810665));
#18937=CARTESIAN_POINT('',(-1.1890923656228,-1.,-0.623405250232602));
#18938=CARTESIAN_POINT('',(-1.1890923656228,-1.,-0.623405250232602));
#18939=CARTESIAN_POINT('',(-1.16272570712099,-1.,-0.6713));
#18940=CARTESIAN_POINT('',(-1.16272570712099,-1.,-0.6713));
#18941=CARTESIAN_POINT('',(-1.13443096636543,-1.,-0.718081570959178));
#18942=CARTESIAN_POINT('',(-1.13443096636543,-1.,-0.718081570959178));
#18943=CARTESIAN_POINT('',(-1.10425506292382,-1.,-0.763672387877889));
#18944=CARTESIAN_POINT('',(-1.10425506292382,-1.,-0.763672387877889));
#18945=CARTESIAN_POINT('',(-1.0722480357895,-1.,-0.80799685008394));
#18946=CARTESIAN_POINT('Origin',(-0.67113967774902,0.,-0.464141716451927));
#18947=CARTESIAN_POINT('',(-0.67113967774902,0.,-0.464141716451927));
#18948=CARTESIAN_POINT('',(-0.651686576198591,0.,-0.491081058892072));
#18949=CARTESIAN_POINT('Origin',(-0.689479866344548,0.,-0.43643271406427));
#18950=CARTESIAN_POINT('',(-0.689479866344548,0.,-0.43643271406427));
#18951=CARTESIAN_POINT('Origin',(-0.706676729488102,0.,-0.408));
#18952=CARTESIAN_POINT('',(-0.706676729488102,0.,-0.408));
#18953=CARTESIAN_POINT('Origin',(-0.722701750594522,0.,-0.378890722620143));
#18954=CARTESIAN_POINT('',(-0.722701750594522,0.,-0.378890722620143));
#18955=CARTESIAN_POINT('Origin',(-0.737528356277993,0.,-0.34915315219239));
#18956=CARTESIAN_POINT('Origin',(-1.21348721953288,0.,-0.574476742810665));
#18957=CARTESIAN_POINT('',(-1.21348721953288,1.,-0.574476742810665));
#18958=CARTESIAN_POINT('',(-1.21348721953288,1.,-0.574476742810665));
#18959=CARTESIAN_POINT('',(-1.21348721953288,0.,-0.574476742810665));
#18960=CARTESIAN_POINT('Origin',(-1.1890923656228,0.,-0.623405250232602));
#18961=CARTESIAN_POINT('',(-1.1890923656228,1.,-0.623405250232602));
#18962=CARTESIAN_POINT('',(-1.1890923656228,1.,-0.623405250232602));
#18963=CARTESIAN_POINT('',(-1.1890923656228,0.,-0.623405250232602));
#18964=CARTESIAN_POINT('Origin',(-1.16272570712099,0.,-0.6713));
#18965=CARTESIAN_POINT('',(-1.16272570712099,1.,-0.6713));
#18966=CARTESIAN_POINT('',(-1.16272570712099,1.,-0.6713));
#18967=CARTESIAN_POINT('',(-1.16272570712099,0.,-0.6713));
#18968=CARTESIAN_POINT('Origin',(-1.13443096636543,0.,-0.718081570959178));
#18969=CARTESIAN_POINT('',(-1.13443096636543,1.,-0.718081570959178));
#18970=CARTESIAN_POINT('',(-1.13443096636543,1.,-0.718081570959178));
#18971=CARTESIAN_POINT('',(-1.13443096636543,0.,-0.718081570959178));
#18972=CARTESIAN_POINT('Origin',(-1.10425506292382,0.,-0.763672387877889));
#18973=CARTESIAN_POINT('',(-1.10425506292382,1.,-0.763672387877889));
#18974=CARTESIAN_POINT('',(-1.10425506292382,1.,-0.763672387877889));
#18975=CARTESIAN_POINT('',(-1.10425506292382,0.,-0.763672387877889));
#18976=CARTESIAN_POINT('Origin',(-1.0722480357895,0.,-0.80799685008394));
#18977=CARTESIAN_POINT('',(-1.0722480357895,1.,-0.80799685008394));
#18978=CARTESIAN_POINT('',(-1.0722480357895,1.,-0.80799685008394));
#18979=CARTESIAN_POINT('',(-1.0722480357895,0.,-0.80799685008394));
#18980=CARTESIAN_POINT('Origin',(-0.651686576198591,0.,-0.491081058892072));
#18981=CARTESIAN_POINT('',(-0.651686576198591,1.,-0.491081058892072));
#18982=CARTESIAN_POINT('Origin',(-0.932067487714439,1.,-0.53812941493483));
#18983=CARTESIAN_POINT('Origin',(0.16362178045575,0.,1.33259246319364));
#18984=CARTESIAN_POINT('',(0.0994453842185998,1.,0.809917659739319));
#18985=CARTESIAN_POINT('',(0.0994453842185998,0.,0.809917659739319));
#18986=CARTESIAN_POINT('',(0.16362178045575,1.,1.33259246319364));
#18987=CARTESIAN_POINT('',(0.16362178045575,1.,1.33259246319364));
#18988=CARTESIAN_POINT('',(0.16362178045575,-1.,1.33259246319364));
#18989=CARTESIAN_POINT('',(0.16362178045575,0.,1.33259246319364));
#18990=CARTESIAN_POINT('',(0.0994453842185998,-1.,0.809917659739319));
#18991=CARTESIAN_POINT('',(0.16362178045575,-1.,1.33259246319364));
#18992=CARTESIAN_POINT('',(0.0994453842185998,0.,0.809917659739319));
#18993=CARTESIAN_POINT('Origin',(0.0994453842185998,0.,0.809917659739319));
#18994=CARTESIAN_POINT('',(0.0663886785289718,1.,0.813294868644317));
#18995=CARTESIAN_POINT('',(0.0663886785289718,0.,0.813294868644317));
#18996=CARTESIAN_POINT('',(0.0994453842185998,1.,0.809917659739319));
#18997=CARTESIAN_POINT('Origin',(0.0994453842185998,0.,0.809917659739319));
#18998=CARTESIAN_POINT('',(0.0663886785289718,-1.,0.813294868644317));
#18999=CARTESIAN_POINT('',(0.0994453842185998,-1.,0.809917659739319));
#19000=CARTESIAN_POINT('',(0.0663886785289718,0.,0.813294868644317));
#19001=CARTESIAN_POINT('Origin',(0.0663886785289718,0.,0.813294868644317));
#19002=CARTESIAN_POINT('',(0.0332218842499737,1.,0.815323436684413));
#19003=CARTESIAN_POINT('',(0.0332218842499737,0.,0.815323436684413));
#19004=CARTESIAN_POINT('',(0.0663886785289718,1.,0.813294868644317));
#19005=CARTESIAN_POINT('Origin',(0.0332218842499737,0.,0.815323436684413));
#19006=CARTESIAN_POINT('',(-4.9960036108132E-16,1.,0.816));
#19007=CARTESIAN_POINT('',(-4.9960036108132E-16,0.,0.816));
#19008=CARTESIAN_POINT('',(0.0332218842499737,1.,0.815323436684413));
#19009=CARTESIAN_POINT('Origin',(-4.9960036108132E-16,0.,0.816));
#19010=CARTESIAN_POINT('',(-0.0332218842499747,1.,0.815323436684413));
#19011=CARTESIAN_POINT('',(-0.0332218842499747,0.,0.815323436684413));
#19012=CARTESIAN_POINT('',(-4.9960036108132E-16,1.,0.816));
#19013=CARTESIAN_POINT('Origin',(-0.0332218842499747,0.,0.815323436684413));
#19014=CARTESIAN_POINT('',(-0.0663886785289729,1.,0.813294868644317));
#19015=CARTESIAN_POINT('',(-0.0663886785289729,0.,0.813294868644317));
#19016=CARTESIAN_POINT('',(-0.0332218842499747,1.,0.815323436684413));
#19017=CARTESIAN_POINT('Origin',(-0.0663886785289729,0.,0.813294868644317));
#19018=CARTESIAN_POINT('',(-0.0994453842186008,1.,0.809917659739319));
#19019=CARTESIAN_POINT('',(-0.0994453842186008,0.,0.809917659739319));
#19020=CARTESIAN_POINT('',(-0.0663886785289729,1.,0.813294868644317));
#19021=CARTESIAN_POINT('Origin',(-6.10622663543836E-16,-1.,1.07625882986966));
#19022=CARTESIAN_POINT('',(-0.163621780455752,-1.,1.33259246319364));
#19023=CARTESIAN_POINT('',(-0.0994453842186008,-1.,0.809917659739319));
#19024=CARTESIAN_POINT('',(-0.0994453842186008,-1.,0.809917659739319));
#19025=CARTESIAN_POINT('',(-0.0663886785289729,-1.,0.813294868644317));
#19026=CARTESIAN_POINT('',(-0.0663886785289729,-1.,0.813294868644317));
#19027=CARTESIAN_POINT('',(-0.0332218842499747,-1.,0.815323436684413));
#19028=CARTESIAN_POINT('',(-0.0332218842499747,-1.,0.815323436684413));
#19029=CARTESIAN_POINT('',(-4.9960036108132E-16,-1.,0.816));
#19030=CARTESIAN_POINT('',(-4.9960036108132E-16,-1.,0.816));
#19031=CARTESIAN_POINT('',(0.0332218842499737,-1.,0.815323436684413));
#19032=CARTESIAN_POINT('',(0.0332218842499737,-1.,0.815323436684413));
#19033=CARTESIAN_POINT('',(0.0663886785289718,-1.,0.813294868644317));
#19034=CARTESIAN_POINT('',(0.109232156609066,-1.,1.33814913068855));
#19035=CARTESIAN_POINT('',(0.109232156609066,-1.,1.33814913068855));
#19036=CARTESIAN_POINT('',(0.054661399257371,-1.,1.34148682119178));
#19037=CARTESIAN_POINT('',(0.054661399257371,-1.,1.34148682119178));
#19038=CARTESIAN_POINT('',(-7.7715611723761E-16,-1.,1.3426));
#19039=CARTESIAN_POINT('',(-7.7715611723761E-16,-1.,1.3426));
#19040=CARTESIAN_POINT('',(-0.0546613992573726,-1.,1.34148682119178));
#19041=CARTESIAN_POINT('',(-0.0546613992573726,-1.,1.34148682119178));
#19042=CARTESIAN_POINT('',(-0.109232156609067,-1.,1.33814913068855));
#19043=CARTESIAN_POINT('',(-0.109232156609067,-1.,1.33814913068855));
#19044=CARTESIAN_POINT('',(-0.163621780455752,-1.,1.33259246319364));
#19045=CARTESIAN_POINT('Origin',(-0.0663886785289729,0.,0.813294868644317));
#19046=CARTESIAN_POINT('',(-0.0663886785289729,0.,0.813294868644317));
#19047=CARTESIAN_POINT('',(-0.0994453842186008,0.,0.809917659739319));
#19048=CARTESIAN_POINT('Origin',(-0.0332218842499747,0.,0.815323436684413));
#19049=CARTESIAN_POINT('',(-0.0332218842499747,0.,0.815323436684413));
#19050=CARTESIAN_POINT('Origin',(-4.9960036108132E-16,0.,0.816));
#19051=CARTESIAN_POINT('',(-4.9960036108132E-16,0.,0.816));
#19052=CARTESIAN_POINT('Origin',(0.0332218842499737,0.,0.815323436684413));
#19053=CARTESIAN_POINT('',(0.0332218842499737,0.,0.815323436684413));
#19054=CARTESIAN_POINT('Origin',(0.0663886785289718,0.,0.813294868644317));
#19055=CARTESIAN_POINT('Origin',(0.109232156609066,0.,1.33814913068855));
#19056=CARTESIAN_POINT('',(0.109232156609066,1.,1.33814913068855));
#19057=CARTESIAN_POINT('',(0.109232156609066,1.,1.33814913068855));
#19058=CARTESIAN_POINT('',(0.109232156609066,0.,1.33814913068855));
#19059=CARTESIAN_POINT('Origin',(0.054661399257371,0.,1.34148682119178));
#19060=CARTESIAN_POINT('',(0.054661399257371,1.,1.34148682119178));
#19061=CARTESIAN_POINT('',(0.054661399257371,1.,1.34148682119178));
#19062=CARTESIAN_POINT('',(0.054661399257371,0.,1.34148682119178));
#19063=CARTESIAN_POINT('Origin',(-7.7715611723761E-16,0.,1.3426));
#19064=CARTESIAN_POINT('',(-7.7715611723761E-16,1.,1.3426));
#19065=CARTESIAN_POINT('',(-7.7715611723761E-16,1.,1.3426));
#19066=CARTESIAN_POINT('',(-7.7715611723761E-16,0.,1.3426));
#19067=CARTESIAN_POINT('Origin',(-0.0546613992573726,0.,1.34148682119178));
#19068=CARTESIAN_POINT('',(-0.0546613992573726,1.,1.34148682119178));
#19069=CARTESIAN_POINT('',(-0.0546613992573726,1.,1.34148682119178));
#19070=CARTESIAN_POINT('',(-0.0546613992573726,0.,1.34148682119178));
#19071=CARTESIAN_POINT('Origin',(-0.109232156609067,0.,1.33814913068855));
#19072=CARTESIAN_POINT('',(-0.109232156609067,1.,1.33814913068855));
#19073=CARTESIAN_POINT('',(-0.109232156609067,1.,1.33814913068855));
#19074=CARTESIAN_POINT('',(-0.109232156609067,0.,1.33814913068855));
#19075=CARTESIAN_POINT('Origin',(-0.163621780455752,0.,1.33259246319364));
#19076=CARTESIAN_POINT('',(-0.163621780455752,1.,1.33259246319364));
#19077=CARTESIAN_POINT('',(-0.163621780455752,1.,1.33259246319364));
#19078=CARTESIAN_POINT('',(-0.163621780455752,0.,1.33259246319364));
#19079=CARTESIAN_POINT('Origin',(-0.0994453842186008,0.,0.809917659739319));
#19080=CARTESIAN_POINT('',(-0.0994453842186008,1.,0.809917659739319));
#19081=CARTESIAN_POINT('Origin',(-6.10622663543836E-16,1.,1.07625882986966));
#19319=UNCERTAINTY_MEASURE_WITH_UNIT(LENGTH_MEASURE(0.001),#19362,
'DISTANCE_ACCURACY_VALUE',
'Maximum model space distance between geometric entities at asserted c
onnectivities');
#19323=UNCERTAINTY_MEASURE_WITH_UNIT(LENGTH_MEASURE(0.001),#19362,
'DISTANCE_ACCURACY_VALUE',
'Maximum model space distance between geometric entities at asserted c
onnectivities');
#19357=(
GEOMETRIC_REPRESENTATION_CONTEXT(3)
GLOBAL_UNCERTAINTY_ASSIGNED_CONTEXT((#19319))
GLOBAL_UNIT_ASSIGNED_CONTEXT((#19362,#19364,#19365))
REPRESENTATION_CONTEXT('','3D')
);
#19361=(
GEOMETRIC_REPRESENTATION_CONTEXT(3)
GLOBAL_UNCERTAINTY_ASSIGNED_CONTEXT((#19323))
GLOBAL_UNIT_ASSIGNED_CONTEXT((#19362,#19364,#19365))
REPRESENTATION_CONTEXT('','3D')
);
#19362=(
LENGTH_UNIT()
NAMED_UNIT(*)
SI_UNIT(.CENTI.,.METRE.)
);
#19364=(
NAMED_UNIT(*)
PLANE_ANGLE_UNIT()
SI_UNIT($,.RADIAN.)
);
#19365=(
NAMED_UNIT(*)
SI_UNIT($,.STERADIAN.)
SOLID_ANGLE_UNIT()
);
#19399=SHAPE_DEFINITION_REPRESENTATION(#19463,#19521);
#19463=PRODUCT_DEFINITION_SHAPE('',$,#19559);
#19521=SHAPE_REPRESENTATION('',(#12100),#19357);
#19525=PRODUCT_DEFINITION_CONTEXT('part definition',#19638,'design');
#19559=PRODUCT_DEFINITION('Spider','Spider',#19596,#19525);
#19596=PRODUCT_DEFINITION_FORMATION('',$,#19673);
#19638=APPLICATION_CONTEXT(
'Core Data for Automotive Mechanical Design Process');
#19639=PRODUCT_CONTEXT('part definition',#19638,'mechanical');
#19673=PRODUCT('Spider','Spider','Spider',(#19639));
#19733=COLOUR_RGB('Sky Blue',0.24,0.69,0.87);
#19734=FILL_AREA_STYLE_COLOUR('',#19733);
#19735=FILL_AREA_STYLE('',(#19734));
#19736=SURFACE_STYLE_FILL_AREA(#19735);
#19737=SURFACE_SIDE_STYLE('',(#19736));
#19738=SURFACE_STYLE_USAGE(.BOTH.,#19737);
#19739=PRESENTATION_STYLE_ASSIGNMENT((#19738));
ENDSEC;
END-ISO-10303-21;
